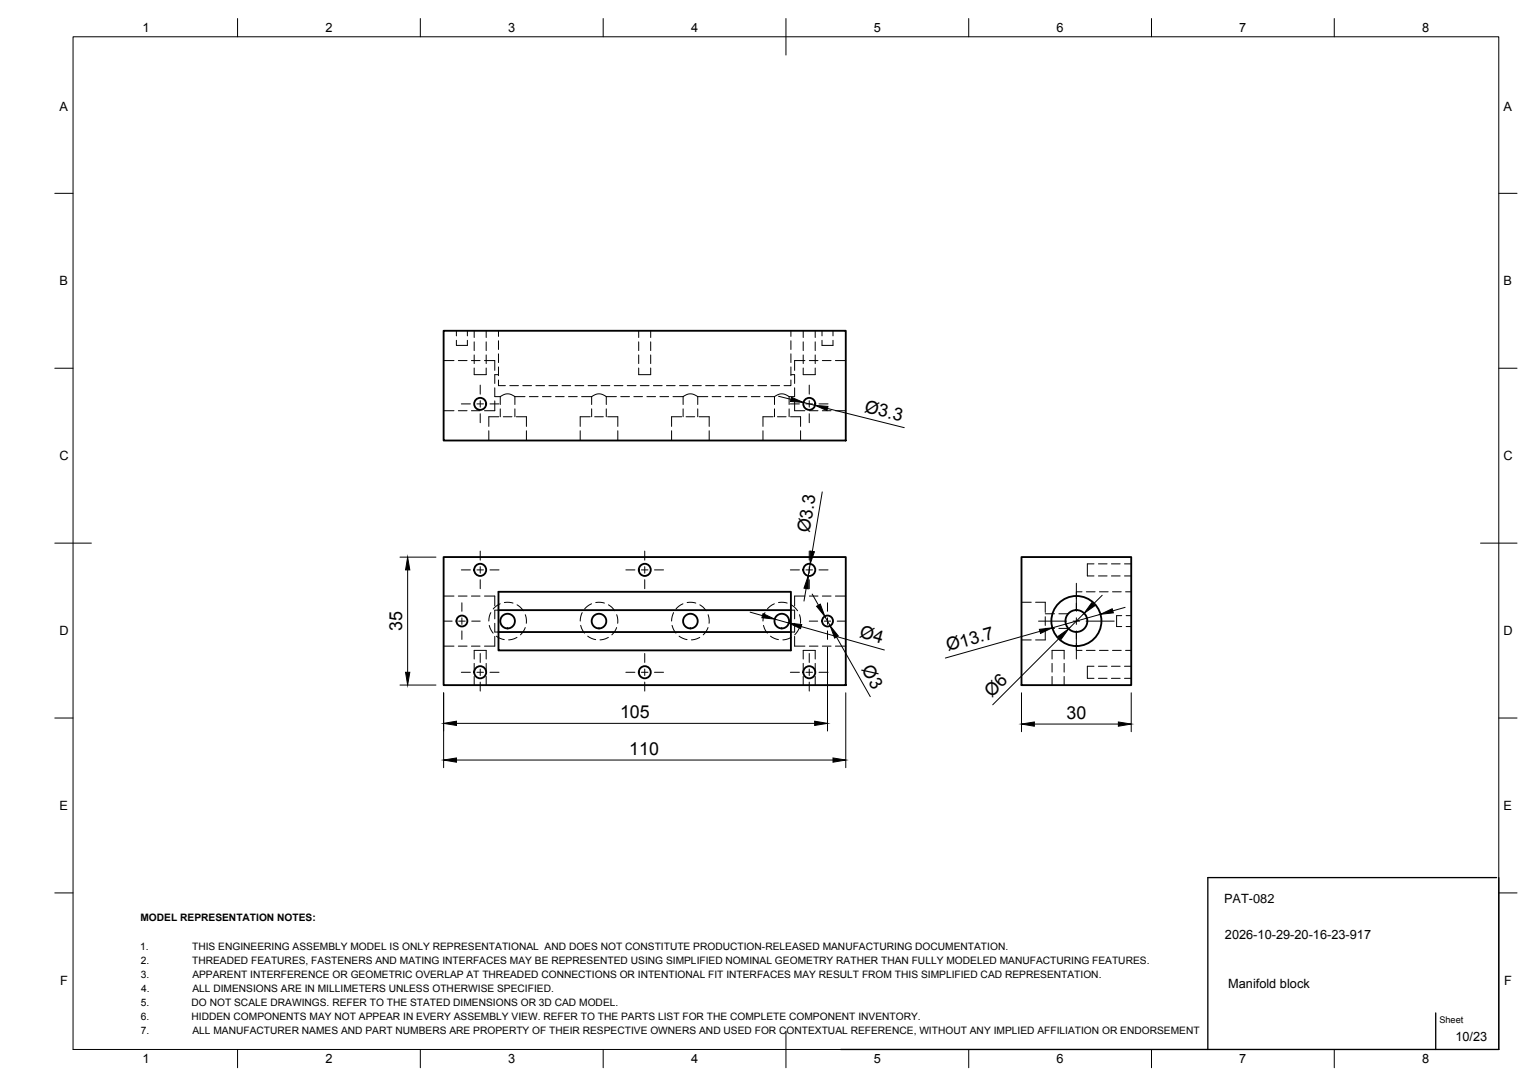
ISO-10303-21;
HEADER;
/* Generated by software containing ST-Developer
 * from STEP Tools, Inc. (www.steptools.com) 
 */

FILE_DESCRIPTION(
/* description */ ('PAT-082'),
/* implementation_level */ '2;1');

FILE_NAME(
/* name */ 'Manifold block.step',
/* time_stamp */ '2026-10-29T20:16:13-07:00',
/* author */ (''),
/* organization */ (''),
/* preprocessor_version */ 'ST-DEVELOPER v20.2',
/* originating_system */ 'Autodesk Translation Framework v15.17.0.0',
/* authorisation */ '');

FILE_SCHEMA (('AUTOMOTIVE_DESIGN { 1 0 10303 214 3 1 1 }'));
ENDSEC;

DATA;
#10=MECHANICAL_DESIGN_GEOMETRIC_PRESENTATION_REPRESENTATION('',(#248),#8266);
#185=B_SPLINE_CURVE_WITH_KNOTS('',3,(#7377,#7378,#7379,#7380,#7381,#7382,
#7383,#7384,#7385,#7386),.UNSPECIFIED.,.F.,.F.,(4,2,2,2,4),(0.,0.0789054703932598,
0.15781094078652,0.235848341776527,0.313885742766535),.UNSPECIFIED.);
#186=B_SPLINE_CURVE_WITH_KNOTS('',3,(#7388,#7389,#7390,#7391,#7392,#7393,
#7394,#7395,#7396,#7397),.UNSPECIFIED.,.F.,.F.,(4,2,2,2,4),(0.941657228299606,
1.01969462928961,1.09773203027962,1.17663750067288,1.25554297106614),
 .UNSPECIFIED.);
#187=B_SPLINE_CURVE_WITH_KNOTS('',3,(#7401,#7402,#7403,#7404,#7405,#7406,
#7407,#7408,#7409,#7410,#7411,#7412,#7413,#7414,#7415,#7416,#7417,#7418),
 .UNSPECIFIED.,.F.,.F.,(4,2,2,2,2,2,2,2,4),(0.313885742766535,0.391923143756543,
0.469960544746551,0.548866015139811,0.627771485533071,0.70667695592633,
0.78558242631959,0.863619827309598,0.941657228299606),.UNSPECIFIED.);
#188=B_SPLINE_CURVE_WITH_KNOTS('',3,(#7429,#7430,#7431,#7432,#7433,#7434,
#7435,#7436,#7437,#7438),.UNSPECIFIED.,.F.,.F.,(4,2,2,2,4),(0.,0.0789054703932594,
0.157810940786519,0.235848341776527,0.313885742766535),.UNSPECIFIED.);
#189=B_SPLINE_CURVE_WITH_KNOTS('',3,(#7440,#7441,#7442,#7443,#7444,#7445,
#7446,#7447,#7448,#7449),.UNSPECIFIED.,.F.,.F.,(4,2,2,2,4),(0.941657228299605,
1.01969462928961,1.09773203027962,1.17663750067288,1.25554297106614),
 .UNSPECIFIED.);
#190=B_SPLINE_CURVE_WITH_KNOTS('',3,(#7453,#7454,#7455,#7456,#7457,#7458,
#7459,#7460,#7461,#7462,#7463,#7464,#7465,#7466,#7467,#7468,#7469,#7470),
 .UNSPECIFIED.,.F.,.F.,(4,2,2,2,2,2,2,2,4),(0.313885742766535,0.391923143756543,
0.46996054474655,0.54886601513981,0.62777148553307,0.70667695592633,0.785582426319589,
0.863619827309597,0.941657228299605),.UNSPECIFIED.);
#191=B_SPLINE_CURVE_WITH_KNOTS('',3,(#7481,#7482,#7483,#7484,#7485,#7486,
#7487,#7488,#7489,#7490),.UNSPECIFIED.,.F.,.F.,(4,2,2,2,4),(0.,0.0789054703932594,
0.157810940786519,0.235848341776527,0.313885742766535),.UNSPECIFIED.);
#192=B_SPLINE_CURVE_WITH_KNOTS('',3,(#7492,#7493,#7494,#7495,#7496,#7497,
#7498,#7499,#7500,#7501),.UNSPECIFIED.,.F.,.F.,(4,2,2,2,4),(0.941657228299605,
1.01969462928961,1.09773203027962,1.17663750067288,1.25554297106614),
 .UNSPECIFIED.);
#193=B_SPLINE_CURVE_WITH_KNOTS('',3,(#7505,#7506,#7507,#7508,#7509,#7510,
#7511,#7512,#7513,#7514,#7515,#7516,#7517,#7518,#7519,#7520,#7521,#7522),
 .UNSPECIFIED.,.F.,.F.,(4,2,2,2,2,2,2,2,4),(0.313885742766535,0.391923143756543,
0.46996054474655,0.54886601513981,0.62777148553307,0.70667695592633,0.785582426319589,
0.863619827309597,0.941657228299605),.UNSPECIFIED.);
#194=B_SPLINE_CURVE_WITH_KNOTS('',3,(#7533,#7534,#7535,#7536,#7537,#7538,
#7539,#7540,#7541,#7542),.UNSPECIFIED.,.F.,.F.,(4,2,2,2,4),(0.,0.0789054703932596,
0.157810940786519,0.235848341776527,0.313885742766535),.UNSPECIFIED.);
#195=B_SPLINE_CURVE_WITH_KNOTS('',3,(#7544,#7545,#7546,#7547,#7548,#7549,
#7550,#7551,#7552,#7553),.UNSPECIFIED.,.F.,.F.,(4,2,2,2,4),(0.941657228299606,
1.01969462928961,1.09773203027962,1.17663750067288,1.25554297106614),
 .UNSPECIFIED.);
#196=B_SPLINE_CURVE_WITH_KNOTS('',3,(#7557,#7558,#7559,#7560,#7561,#7562,
#7563,#7564,#7565,#7566,#7567,#7568,#7569,#7570,#7571,#7572,#7573,#7574),
 .UNSPECIFIED.,.F.,.F.,(4,2,2,2,2,2,2,2,4),(0.313885742766535,0.391923143756543,
0.469960544746551,0.548866015139811,0.62777148553307,0.70667695592633,0.78558242631959,
0.863619827309598,0.941657228299606),.UNSPECIFIED.);
#204=SHAPE_REPRESENTATION_RELATIONSHIP('SRR','None',#8366,#226);
#226=ADVANCED_BREP_SHAPE_REPRESENTATION('',(#270),#8250);
#248=STYLED_ITEM('',(#8516),#270);
#270=MANIFOLD_SOLID_BREP('Body1',#4588);
#352=FACE_BOUND('',#1028,.T.);
#353=FACE_BOUND('',#1031,.T.);
#354=FACE_BOUND('',#1035,.T.);
#355=FACE_BOUND('',#1039,.T.);
#356=FACE_BOUND('',#1043,.T.);
#357=FACE_BOUND('',#1047,.T.);
#358=FACE_BOUND('',#1055,.T.);
#359=FACE_BOUND('',#1058,.T.);
#360=FACE_BOUND('',#1060,.T.);
#361=FACE_BOUND('',#1061,.T.);
#362=FACE_BOUND('',#1063,.T.);
#363=FACE_BOUND('',#1065,.T.);
#364=FACE_BOUND('',#1066,.T.);
#365=FACE_BOUND('',#1067,.T.);
#366=FACE_BOUND('',#1068,.T.);
#367=FACE_BOUND('',#1070,.T.);
#368=FACE_BOUND('',#1071,.T.);
#369=FACE_BOUND('',#1072,.T.);
#370=FACE_BOUND('',#1073,.T.);
#371=FACE_BOUND('',#1074,.T.);
#372=FACE_BOUND('',#1075,.T.);
#373=FACE_BOUND('',#1076,.T.);
#374=FACE_BOUND('',#1077,.T.);
#375=FACE_BOUND('',#1078,.T.);
#459=PLANE('',#5043);
#460=PLANE('',#5047);
#461=PLANE('',#5051);
#462=PLANE('',#5055);
#463=PLANE('',#5059);
#464=PLANE('',#5063);
#465=PLANE('',#5067);
#466=PLANE('',#5071);
#467=PLANE('',#5075);
#468=PLANE('',#5079);
#469=PLANE('',#5083);
#470=PLANE('',#5088);
#471=PLANE('',#5095);
#472=PLANE('',#5101);
#473=PLANE('',#5107);
#474=PLANE('',#5113);
#475=PLANE('',#5114);
#476=PLANE('',#5115);
#477=PLANE('',#5117);
#478=PLANE('',#5118);
#479=PLANE('',#5119);
#480=PLANE('',#5121);
#481=PLANE('',#5123);
#482=PLANE('',#5124);
#483=PLANE('',#5125);
#484=PLANE('',#5126);
#485=PLANE('',#5127);
#486=PLANE('',#5128);
#666=FACE_OUTER_BOUND('',#1006,.T.);
#667=FACE_OUTER_BOUND('',#1007,.T.);
#668=FACE_OUTER_BOUND('',#1008,.T.);
#669=FACE_OUTER_BOUND('',#1009,.T.);
#670=FACE_OUTER_BOUND('',#1010,.T.);
#671=FACE_OUTER_BOUND('',#1011,.T.);
#672=FACE_OUTER_BOUND('',#1012,.T.);
#673=FACE_OUTER_BOUND('',#1013,.T.);
#674=FACE_OUTER_BOUND('',#1014,.T.);
#675=FACE_OUTER_BOUND('',#1015,.T.);
#676=FACE_OUTER_BOUND('',#1016,.T.);
#677=FACE_OUTER_BOUND('',#1017,.T.);
#678=FACE_OUTER_BOUND('',#1018,.T.);
#679=FACE_OUTER_BOUND('',#1019,.T.);
#680=FACE_OUTER_BOUND('',#1020,.T.);
#681=FACE_OUTER_BOUND('',#1021,.T.);
#682=FACE_OUTER_BOUND('',#1022,.T.);
#683=FACE_OUTER_BOUND('',#1023,.T.);
#684=FACE_OUTER_BOUND('',#1024,.T.);
#685=FACE_OUTER_BOUND('',#1025,.T.);
#686=FACE_OUTER_BOUND('',#1026,.T.);
#687=FACE_OUTER_BOUND('',#1027,.T.);
#688=FACE_OUTER_BOUND('',#1029,.T.);
#689=FACE_OUTER_BOUND('',#1030,.T.);
#690=FACE_OUTER_BOUND('',#1032,.T.);
#691=FACE_OUTER_BOUND('',#1033,.T.);
#692=FACE_OUTER_BOUND('',#1034,.T.);
#693=FACE_OUTER_BOUND('',#1036,.T.);
#694=FACE_OUTER_BOUND('',#1037,.T.);
#695=FACE_OUTER_BOUND('',#1038,.T.);
#696=FACE_OUTER_BOUND('',#1040,.T.);
#697=FACE_OUTER_BOUND('',#1041,.T.);
#698=FACE_OUTER_BOUND('',#1042,.T.);
#699=FACE_OUTER_BOUND('',#1044,.T.);
#700=FACE_OUTER_BOUND('',#1045,.T.);
#701=FACE_OUTER_BOUND('',#1046,.T.);
#702=FACE_OUTER_BOUND('',#1048,.T.);
#703=FACE_OUTER_BOUND('',#1049,.T.);
#704=FACE_OUTER_BOUND('',#1050,.T.);
#705=FACE_OUTER_BOUND('',#1051,.T.);
#706=FACE_OUTER_BOUND('',#1052,.T.);
#707=FACE_OUTER_BOUND('',#1053,.T.);
#708=FACE_OUTER_BOUND('',#1054,.T.);
#709=FACE_OUTER_BOUND('',#1056,.T.);
#710=FACE_OUTER_BOUND('',#1057,.T.);
#711=FACE_OUTER_BOUND('',#1059,.T.);
#712=FACE_OUTER_BOUND('',#1062,.T.);
#713=FACE_OUTER_BOUND('',#1064,.T.);
#714=FACE_OUTER_BOUND('',#1069,.T.);
#1006=EDGE_LOOP('',(#3542,#3543,#3544,#3545));
#1007=EDGE_LOOP('',(#3546));
#1008=EDGE_LOOP('',(#3547,#3548,#3549,#3550));
#1009=EDGE_LOOP('',(#3551));
#1010=EDGE_LOOP('',(#3552,#3553,#3554,#3555));
#1011=EDGE_LOOP('',(#3556));
#1012=EDGE_LOOP('',(#3557,#3558,#3559,#3560));
#1013=EDGE_LOOP('',(#3561));
#1014=EDGE_LOOP('',(#3562,#3563,#3564,#3565));
#1015=EDGE_LOOP('',(#3566));
#1016=EDGE_LOOP('',(#3567,#3568,#3569,#3570));
#1017=EDGE_LOOP('',(#3571));
#1018=EDGE_LOOP('',(#3572,#3573,#3574,#3575));
#1019=EDGE_LOOP('',(#3576));
#1020=EDGE_LOOP('',(#3577,#3578,#3579,#3580));
#1021=EDGE_LOOP('',(#3581));
#1022=EDGE_LOOP('',(#3582,#3583,#3584,#3585));
#1023=EDGE_LOOP('',(#3586));
#1024=EDGE_LOOP('',(#3587,#3588,#3589,#3590));
#1025=EDGE_LOOP('',(#3591));
#1026=EDGE_LOOP('',(#3592,#3593,#3594,#3595));
#1027=EDGE_LOOP('',(#3596));
#1028=EDGE_LOOP('',(#3597));
#1029=EDGE_LOOP('',(#3598,#3599,#3600,#3601));
#1030=EDGE_LOOP('',(#3602));
#1031=EDGE_LOOP('',(#3603));
#1032=EDGE_LOOP('',(#3604,#3605,#3606,#3607,#3608,#3609));
#1033=EDGE_LOOP('',(#3610,#3611,#3612,#3613));
#1034=EDGE_LOOP('',(#3614));
#1035=EDGE_LOOP('',(#3615));
#1036=EDGE_LOOP('',(#3616,#3617,#3618,#3619,#3620,#3621));
#1037=EDGE_LOOP('',(#3622,#3623,#3624,#3625));
#1038=EDGE_LOOP('',(#3626));
#1039=EDGE_LOOP('',(#3627));
#1040=EDGE_LOOP('',(#3628,#3629,#3630,#3631,#3632,#3633));
#1041=EDGE_LOOP('',(#3634,#3635,#3636,#3637));
#1042=EDGE_LOOP('',(#3638));
#1043=EDGE_LOOP('',(#3639));
#1044=EDGE_LOOP('',(#3640,#3641,#3642,#3643,#3644,#3645));
#1045=EDGE_LOOP('',(#3646,#3647,#3648,#3649));
#1046=EDGE_LOOP('',(#3650));
#1047=EDGE_LOOP('',(#3651));
#1048=EDGE_LOOP('',(#3652,#3653,#3654,#3655));
#1049=EDGE_LOOP('',(#3656,#3657,#3658,#3659,#3660,#3661));
#1050=EDGE_LOOP('',(#3662,#3663,#3664,#3665));
#1051=EDGE_LOOP('',(#3666,#3667,#3668,#3669));
#1052=EDGE_LOOP('',(#3670,#3671,#3672,#3673,#3674,#3675));
#1053=EDGE_LOOP('',(#3676,#3677,#3678,#3679));
#1054=EDGE_LOOP('',(#3680,#3681,#3682,#3683,#3684,#3685,#3686,#3687,#3688,
#3689,#3690,#3691,#3692,#3693,#3694,#3695,#3696,#3697,#3698,#3699,#3700,
#3701,#3702,#3703));
#1055=EDGE_LOOP('',(#3704,#3705,#3706,#3707));
#1056=EDGE_LOOP('',(#3708,#3709,#3710,#3711));
#1057=EDGE_LOOP('',(#3712,#3713,#3714,#3715));
#1058=EDGE_LOOP('',(#3716));
#1059=EDGE_LOOP('',(#3717,#3718,#3719,#3720));
#1060=EDGE_LOOP('',(#3721));
#1061=EDGE_LOOP('',(#3722));
#1062=EDGE_LOOP('',(#3723,#3724,#3725,#3726));
#1063=EDGE_LOOP('',(#3727));
#1064=EDGE_LOOP('',(#3728,#3729,#3730,#3731));
#1065=EDGE_LOOP('',(#3732));
#1066=EDGE_LOOP('',(#3733));
#1067=EDGE_LOOP('',(#3734));
#1068=EDGE_LOOP('',(#3735));
#1069=EDGE_LOOP('',(#3736,#3737,#3738,#3739));
#1070=EDGE_LOOP('',(#3740));
#1071=EDGE_LOOP('',(#3741,#3742,#3743,#3744));
#1072=EDGE_LOOP('',(#3745));
#1073=EDGE_LOOP('',(#3746));
#1074=EDGE_LOOP('',(#3747));
#1075=EDGE_LOOP('',(#3748));
#1076=EDGE_LOOP('',(#3749));
#1077=EDGE_LOOP('',(#3750));
#1078=EDGE_LOOP('',(#3751));
#1375=LINE('',#7290,#1730);
#1376=LINE('',#7297,#1731);
#1377=LINE('',#7304,#1732);
#1378=LINE('',#7311,#1733);
#1379=LINE('',#7318,#1734);
#1380=LINE('',#7325,#1735);
#1381=LINE('',#7332,#1736);
#1382=LINE('',#7339,#1737);
#1383=LINE('',#7346,#1738);
#1384=LINE('',#7353,#1739);
#1385=LINE('',#7360,#1740);
#1386=LINE('',#7369,#1741);
#1387=LINE('',#7399,#1742);
#1388=LINE('',#7423,#1743);
#1389=LINE('',#7451,#1744);
#1390=LINE('',#7475,#1745);
#1391=LINE('',#7503,#1746);
#1392=LINE('',#7527,#1747);
#1393=LINE('',#7555,#1748);
#1394=LINE('',#7579,#1749);
#1395=LINE('',#7585,#1750);
#1396=LINE('',#7587,#1751);
#1397=LINE('',#7589,#1752);
#1398=LINE('',#7590,#1753);
#1399=LINE('',#7593,#1754);
#1400=LINE('',#7595,#1755);
#1401=LINE('',#7599,#1756);
#1402=LINE('',#7600,#1757);
#1403=LINE('',#7603,#1758);
#1404=LINE('',#7604,#1759);
#1405=LINE('',#7607,#1760);
#1406=LINE('',#7609,#1761);
#1407=LINE('',#7610,#1762);
#1408=LINE('',#7612,#1763);
#1409=LINE('',#7614,#1764);
#1410=LINE('',#7617,#1765);
#1411=LINE('',#7619,#1766);
#1412=LINE('',#7620,#1767);
#1413=LINE('',#7621,#1768);
#1414=LINE('',#7622,#1769);
#1415=LINE('',#7623,#1770);
#1416=LINE('',#7627,#1771);
#1417=LINE('',#7629,#1772);
#1418=LINE('',#7631,#1773);
#1419=LINE('',#7632,#1774);
#1420=LINE('',#7635,#1775);
#1421=LINE('',#7637,#1776);
#1422=LINE('',#7638,#1777);
#1423=LINE('',#7641,#1778);
#1424=LINE('',#7643,#1779);
#1425=LINE('',#7644,#1780);
#1426=LINE('',#7646,#1781);
#1427=LINE('',#7647,#1782);
#1730=VECTOR('',#5908,0.165);
#1731=VECTOR('',#5917,0.165);
#1732=VECTOR('',#5926,0.15);
#1733=VECTOR('',#5935,0.15);
#1734=VECTOR('',#5944,0.165);
#1735=VECTOR('',#5953,0.165);
#1736=VECTOR('',#5962,0.165);
#1737=VECTOR('',#5971,0.165);
#1738=VECTOR('',#5980,0.165);
#1739=VECTOR('',#5989,0.165);
#1740=VECTOR('',#5998,0.685);
#1741=VECTOR('',#6009,0.685);
#1742=VECTOR('',#6018,0.2);
#1743=VECTOR('',#6025,0.515);
#1744=VECTOR('',#6032,0.2);
#1745=VECTOR('',#6039,0.515);
#1746=VECTOR('',#6046,0.2);
#1747=VECTOR('',#6053,0.515);
#1748=VECTOR('',#6060,0.2);
#1749=VECTOR('',#6067,0.515);
#1750=VECTOR('',#6074,1.);
#1751=VECTOR('',#6075,1.);
#1752=VECTOR('',#6076,1.);
#1753=VECTOR('',#6077,1.);
#1754=VECTOR('',#6080,1.);
#1755=VECTOR('',#6081,1.);
#1756=VECTOR('',#6084,1.);
#1757=VECTOR('',#6085,1.);
#1758=VECTOR('',#6088,1.);
#1759=VECTOR('',#6089,1.);
#1760=VECTOR('',#6092,1.);
#1761=VECTOR('',#6093,1.);
#1762=VECTOR('',#6094,1.);
#1763=VECTOR('',#6097,1.);
#1764=VECTOR('',#6098,1.);
#1765=VECTOR('',#6103,1.);
#1766=VECTOR('',#6106,0.3);
#1767=VECTOR('',#6107,0.3);
#1768=VECTOR('',#6108,0.3);
#1769=VECTOR('',#6109,0.3);
#1770=VECTOR('',#6110,0.3);
#1771=VECTOR('',#6113,1.);
#1772=VECTOR('',#6114,1.);
#1773=VECTOR('',#6115,1.);
#1774=VECTOR('',#6116,1.);
#1775=VECTOR('',#6119,1.);
#1776=VECTOR('',#6120,1.);
#1777=VECTOR('',#6121,1.);
#1778=VECTOR('',#6124,1.);
#1779=VECTOR('',#6125,1.);
#1780=VECTOR('',#6126,1.);
#1781=VECTOR('',#6129,1.);
#1782=VECTOR('',#6130,1.);
#2033=CIRCLE('',#5041,0.165);
#2034=CIRCLE('',#5042,0.165);
#2035=CIRCLE('',#5045,0.165);
#2036=CIRCLE('',#5046,0.165);
#2037=CIRCLE('',#5049,0.15);
#2038=CIRCLE('',#5050,0.15);
#2039=CIRCLE('',#5053,0.15);
#2040=CIRCLE('',#5054,0.15);
#2041=CIRCLE('',#5057,0.165);
#2042=CIRCLE('',#5058,0.165);
#2043=CIRCLE('',#5061,0.165);
#2044=CIRCLE('',#5062,0.165);
#2045=CIRCLE('',#5065,0.165);
#2046=CIRCLE('',#5066,0.165);
#2047=CIRCLE('',#5069,0.165);
#2048=CIRCLE('',#5070,0.165);
#2049=CIRCLE('',#5073,0.165);
#2050=CIRCLE('',#5074,0.165);
#2051=CIRCLE('',#5077,0.165);
#2052=CIRCLE('',#5078,0.165);
#2053=CIRCLE('',#5081,0.685);
#2054=CIRCLE('',#5082,0.685);
#2055=CIRCLE('',#5084,0.3);
#2056=CIRCLE('',#5086,0.685);
#2057=CIRCLE('',#5087,0.685);
#2058=CIRCLE('',#5089,0.3);
#2059=CIRCLE('',#5091,0.2);
#2060=CIRCLE('',#5093,0.515);
#2061=CIRCLE('',#5094,0.515);
#2062=CIRCLE('',#5097,0.2);
#2063=CIRCLE('',#5099,0.515);
#2064=CIRCLE('',#5100,0.515);
#2065=CIRCLE('',#5103,0.2);
#2066=CIRCLE('',#5105,0.515);
#2067=CIRCLE('',#5106,0.515);
#2068=CIRCLE('',#5109,0.2);
#2069=CIRCLE('',#5111,0.515);
#2070=CIRCLE('',#5112,0.515);
#2071=CIRCLE('',#5116,0.3);
#2072=CIRCLE('',#5120,0.3);
#2297=VERTEX_POINT('',#7287);
#2298=VERTEX_POINT('',#7289);
#2299=VERTEX_POINT('',#7294);
#2300=VERTEX_POINT('',#7296);
#2301=VERTEX_POINT('',#7301);
#2302=VERTEX_POINT('',#7303);
#2303=VERTEX_POINT('',#7308);
#2304=VERTEX_POINT('',#7310);
#2305=VERTEX_POINT('',#7315);
#2306=VERTEX_POINT('',#7317);
#2307=VERTEX_POINT('',#7322);
#2308=VERTEX_POINT('',#7324);
#2309=VERTEX_POINT('',#7329);
#2310=VERTEX_POINT('',#7331);
#2311=VERTEX_POINT('',#7336);
#2312=VERTEX_POINT('',#7338);
#2313=VERTEX_POINT('',#7343);
#2314=VERTEX_POINT('',#7345);
#2315=VERTEX_POINT('',#7350);
#2316=VERTEX_POINT('',#7352);
#2317=VERTEX_POINT('',#7357);
#2318=VERTEX_POINT('',#7359);
#2319=VERTEX_POINT('',#7363);
#2320=VERTEX_POINT('',#7366);
#2321=VERTEX_POINT('',#7368);
#2322=VERTEX_POINT('',#7372);
#2323=VERTEX_POINT('',#7375);
#2324=VERTEX_POINT('',#7376);
#2325=VERTEX_POINT('',#7387);
#2326=VERTEX_POINT('',#7398);
#2327=VERTEX_POINT('',#7420);
#2328=VERTEX_POINT('',#7422);
#2329=VERTEX_POINT('',#7427);
#2330=VERTEX_POINT('',#7428);
#2331=VERTEX_POINT('',#7439);
#2332=VERTEX_POINT('',#7450);
#2333=VERTEX_POINT('',#7472);
#2334=VERTEX_POINT('',#7474);
#2335=VERTEX_POINT('',#7479);
#2336=VERTEX_POINT('',#7480);
#2337=VERTEX_POINT('',#7491);
#2338=VERTEX_POINT('',#7502);
#2339=VERTEX_POINT('',#7524);
#2340=VERTEX_POINT('',#7526);
#2341=VERTEX_POINT('',#7531);
#2342=VERTEX_POINT('',#7532);
#2343=VERTEX_POINT('',#7543);
#2344=VERTEX_POINT('',#7554);
#2345=VERTEX_POINT('',#7576);
#2346=VERTEX_POINT('',#7578);
#2347=VERTEX_POINT('',#7583);
#2348=VERTEX_POINT('',#7584);
#2349=VERTEX_POINT('',#7586);
#2350=VERTEX_POINT('',#7588);
#2351=VERTEX_POINT('',#7592);
#2352=VERTEX_POINT('',#7594);
#2353=VERTEX_POINT('',#7596);
#2354=VERTEX_POINT('',#7598);
#2355=VERTEX_POINT('',#7602);
#2356=VERTEX_POINT('',#7606);
#2357=VERTEX_POINT('',#7608);
#2358=VERTEX_POINT('',#7613);
#2359=VERTEX_POINT('',#7625);
#2360=VERTEX_POINT('',#7626);
#2361=VERTEX_POINT('',#7628);
#2362=VERTEX_POINT('',#7630);
#2363=VERTEX_POINT('',#7634);
#2364=VERTEX_POINT('',#7636);
#2365=VERTEX_POINT('',#7640);
#2366=VERTEX_POINT('',#7642);
#2747=EDGE_CURVE('',#2297,#2297,#2033,.T.);
#2748=EDGE_CURVE('',#2297,#2298,#1375,.T.);
#2749=EDGE_CURVE('',#2298,#2298,#2034,.T.);
#2750=EDGE_CURVE('',#2299,#2299,#2035,.T.);
#2751=EDGE_CURVE('',#2299,#2300,#1376,.T.);
#2752=EDGE_CURVE('',#2300,#2300,#2036,.T.);
#2753=EDGE_CURVE('',#2301,#2301,#2037,.T.);
#2754=EDGE_CURVE('',#2301,#2302,#1377,.T.);
#2755=EDGE_CURVE('',#2302,#2302,#2038,.T.);
#2756=EDGE_CURVE('',#2303,#2303,#2039,.T.);
#2757=EDGE_CURVE('',#2303,#2304,#1378,.T.);
#2758=EDGE_CURVE('',#2304,#2304,#2040,.T.);
#2759=EDGE_CURVE('',#2305,#2305,#2041,.T.);
#2760=EDGE_CURVE('',#2305,#2306,#1379,.T.);
#2761=EDGE_CURVE('',#2306,#2306,#2042,.T.);
#2762=EDGE_CURVE('',#2307,#2307,#2043,.T.);
#2763=EDGE_CURVE('',#2307,#2308,#1380,.T.);
#2764=EDGE_CURVE('',#2308,#2308,#2044,.T.);
#2765=EDGE_CURVE('',#2309,#2309,#2045,.T.);
#2766=EDGE_CURVE('',#2309,#2310,#1381,.T.);
#2767=EDGE_CURVE('',#2310,#2310,#2046,.T.);
#2768=EDGE_CURVE('',#2311,#2311,#2047,.T.);
#2769=EDGE_CURVE('',#2311,#2312,#1382,.T.);
#2770=EDGE_CURVE('',#2312,#2312,#2048,.T.);
#2771=EDGE_CURVE('',#2313,#2313,#2049,.T.);
#2772=EDGE_CURVE('',#2313,#2314,#1383,.T.);
#2773=EDGE_CURVE('',#2314,#2314,#2050,.T.);
#2774=EDGE_CURVE('',#2315,#2315,#2051,.T.);
#2775=EDGE_CURVE('',#2315,#2316,#1384,.T.);
#2776=EDGE_CURVE('',#2316,#2316,#2052,.T.);
#2777=EDGE_CURVE('',#2317,#2317,#2053,.T.);
#2778=EDGE_CURVE('',#2317,#2318,#1385,.T.);
#2779=EDGE_CURVE('',#2318,#2318,#2054,.T.);
#2780=EDGE_CURVE('',#2319,#2319,#2055,.T.);
#2781=EDGE_CURVE('',#2320,#2320,#2056,.T.);
#2782=EDGE_CURVE('',#2320,#2321,#1386,.T.);
#2783=EDGE_CURVE('',#2321,#2321,#2057,.T.);
#2784=EDGE_CURVE('',#2322,#2322,#2058,.T.);
#2785=EDGE_CURVE('',#2323,#2324,#185,.T.);
#2786=EDGE_CURVE('',#2325,#2323,#186,.T.);
#2787=EDGE_CURVE('',#2325,#2326,#1387,.T.);
#2788=EDGE_CURVE('',#2326,#2326,#2059,.T.);
#2789=EDGE_CURVE('',#2324,#2325,#187,.T.);
#2790=EDGE_CURVE('',#2327,#2327,#2060,.T.);
#2791=EDGE_CURVE('',#2327,#2328,#1388,.T.);
#2792=EDGE_CURVE('',#2328,#2328,#2061,.T.);
#2793=EDGE_CURVE('',#2329,#2330,#188,.T.);
#2794=EDGE_CURVE('',#2331,#2329,#189,.T.);
#2795=EDGE_CURVE('',#2331,#2332,#1389,.T.);
#2796=EDGE_CURVE('',#2332,#2332,#2062,.T.);
#2797=EDGE_CURVE('',#2330,#2331,#190,.T.);
#2798=EDGE_CURVE('',#2333,#2333,#2063,.T.);
#2799=EDGE_CURVE('',#2333,#2334,#1390,.T.);
#2800=EDGE_CURVE('',#2334,#2334,#2064,.T.);
#2801=EDGE_CURVE('',#2335,#2336,#191,.T.);
#2802=EDGE_CURVE('',#2337,#2335,#192,.T.);
#2803=EDGE_CURVE('',#2337,#2338,#1391,.T.);
#2804=EDGE_CURVE('',#2338,#2338,#2065,.T.);
#2805=EDGE_CURVE('',#2336,#2337,#193,.T.);
#2806=EDGE_CURVE('',#2339,#2339,#2066,.T.);
#2807=EDGE_CURVE('',#2339,#2340,#1392,.T.);
#2808=EDGE_CURVE('',#2340,#2340,#2067,.T.);
#2809=EDGE_CURVE('',#2341,#2342,#194,.T.);
#2810=EDGE_CURVE('',#2343,#2341,#195,.T.);
#2811=EDGE_CURVE('',#2343,#2344,#1393,.T.);
#2812=EDGE_CURVE('',#2344,#2344,#2068,.T.);
#2813=EDGE_CURVE('',#2342,#2343,#196,.T.);
#2814=EDGE_CURVE('',#2345,#2345,#2069,.T.);
#2815=EDGE_CURVE('',#2345,#2346,#1394,.T.);
#2816=EDGE_CURVE('',#2346,#2346,#2070,.T.);
#2817=EDGE_CURVE('',#2347,#2348,#1395,.T.);
#2818=EDGE_CURVE('',#2347,#2349,#1396,.T.);
#2819=EDGE_CURVE('',#2349,#2350,#1397,.T.);
#2820=EDGE_CURVE('',#2348,#2350,#1398,.T.);
#2821=EDGE_CURVE('',#2348,#2351,#1399,.T.);
#2822=EDGE_CURVE('',#2350,#2352,#1400,.T.);
#2823=EDGE_CURVE('',#2353,#2352,#2071,.T.);
#2824=EDGE_CURVE('',#2353,#2354,#1401,.T.);
#2825=EDGE_CURVE('',#2351,#2354,#1402,.T.);
#2826=EDGE_CURVE('',#2352,#2355,#1403,.T.);
#2827=EDGE_CURVE('',#2355,#2349,#1404,.T.);
#2828=EDGE_CURVE('',#2351,#2356,#1405,.T.);
#2829=EDGE_CURVE('',#2354,#2357,#1406,.T.);
#2830=EDGE_CURVE('',#2356,#2357,#1407,.T.);
#2831=EDGE_CURVE('',#2356,#2347,#1408,.T.);
#2832=EDGE_CURVE('',#2357,#2358,#1409,.T.);
#2833=EDGE_CURVE('',#2355,#2358,#2072,.T.);
#2834=EDGE_CURVE('',#2358,#2353,#1410,.T.);
#2835=EDGE_CURVE('',#2322,#2343,#1411,.T.);
#2836=EDGE_CURVE('',#2342,#2337,#1412,.T.);
#2837=EDGE_CURVE('',#2336,#2331,#1413,.T.);
#2838=EDGE_CURVE('',#2330,#2325,#1414,.T.);
#2839=EDGE_CURVE('',#2324,#2319,#1415,.T.);
#2840=EDGE_CURVE('',#2359,#2360,#1416,.T.);
#2841=EDGE_CURVE('',#2360,#2361,#1417,.T.);
#2842=EDGE_CURVE('',#2362,#2361,#1418,.T.);
#2843=EDGE_CURVE('',#2359,#2362,#1419,.T.);
#2844=EDGE_CURVE('',#2363,#2359,#1420,.T.);
#2845=EDGE_CURVE('',#2364,#2362,#1421,.T.);
#2846=EDGE_CURVE('',#2363,#2364,#1422,.T.);
#2847=EDGE_CURVE('',#2365,#2363,#1423,.T.);
#2848=EDGE_CURVE('',#2366,#2364,#1424,.T.);
#2849=EDGE_CURVE('',#2365,#2366,#1425,.T.);
#2850=EDGE_CURVE('',#2360,#2365,#1426,.T.);
#2851=EDGE_CURVE('',#2361,#2366,#1427,.T.);
#3542=ORIENTED_EDGE('',*,*,#2747,.F.);
#3543=ORIENTED_EDGE('',*,*,#2748,.T.);
#3544=ORIENTED_EDGE('',*,*,#2749,.T.);
#3545=ORIENTED_EDGE('',*,*,#2748,.F.);
#3546=ORIENTED_EDGE('',*,*,#2749,.F.);
#3547=ORIENTED_EDGE('',*,*,#2750,.F.);
#3548=ORIENTED_EDGE('',*,*,#2751,.T.);
#3549=ORIENTED_EDGE('',*,*,#2752,.T.);
#3550=ORIENTED_EDGE('',*,*,#2751,.F.);
#3551=ORIENTED_EDGE('',*,*,#2752,.F.);
#3552=ORIENTED_EDGE('',*,*,#2753,.F.);
#3553=ORIENTED_EDGE('',*,*,#2754,.T.);
#3554=ORIENTED_EDGE('',*,*,#2755,.T.);
#3555=ORIENTED_EDGE('',*,*,#2754,.F.);
#3556=ORIENTED_EDGE('',*,*,#2755,.F.);
#3557=ORIENTED_EDGE('',*,*,#2756,.F.);
#3558=ORIENTED_EDGE('',*,*,#2757,.T.);
#3559=ORIENTED_EDGE('',*,*,#2758,.T.);
#3560=ORIENTED_EDGE('',*,*,#2757,.F.);
#3561=ORIENTED_EDGE('',*,*,#2758,.F.);
#3562=ORIENTED_EDGE('',*,*,#2759,.F.);
#3563=ORIENTED_EDGE('',*,*,#2760,.T.);
#3564=ORIENTED_EDGE('',*,*,#2761,.T.);
#3565=ORIENTED_EDGE('',*,*,#2760,.F.);
#3566=ORIENTED_EDGE('',*,*,#2761,.F.);
#3567=ORIENTED_EDGE('',*,*,#2762,.F.);
#3568=ORIENTED_EDGE('',*,*,#2763,.T.);
#3569=ORIENTED_EDGE('',*,*,#2764,.T.);
#3570=ORIENTED_EDGE('',*,*,#2763,.F.);
#3571=ORIENTED_EDGE('',*,*,#2764,.F.);
#3572=ORIENTED_EDGE('',*,*,#2765,.F.);
#3573=ORIENTED_EDGE('',*,*,#2766,.T.);
#3574=ORIENTED_EDGE('',*,*,#2767,.T.);
#3575=ORIENTED_EDGE('',*,*,#2766,.F.);
#3576=ORIENTED_EDGE('',*,*,#2767,.F.);
#3577=ORIENTED_EDGE('',*,*,#2768,.F.);
#3578=ORIENTED_EDGE('',*,*,#2769,.T.);
#3579=ORIENTED_EDGE('',*,*,#2770,.T.);
#3580=ORIENTED_EDGE('',*,*,#2769,.F.);
#3581=ORIENTED_EDGE('',*,*,#2770,.F.);
#3582=ORIENTED_EDGE('',*,*,#2771,.F.);
#3583=ORIENTED_EDGE('',*,*,#2772,.T.);
#3584=ORIENTED_EDGE('',*,*,#2773,.T.);
#3585=ORIENTED_EDGE('',*,*,#2772,.F.);
#3586=ORIENTED_EDGE('',*,*,#2773,.F.);
#3587=ORIENTED_EDGE('',*,*,#2774,.F.);
#3588=ORIENTED_EDGE('',*,*,#2775,.T.);
#3589=ORIENTED_EDGE('',*,*,#2776,.T.);
#3590=ORIENTED_EDGE('',*,*,#2775,.F.);
#3591=ORIENTED_EDGE('',*,*,#2776,.F.);
#3592=ORIENTED_EDGE('',*,*,#2777,.F.);
#3593=ORIENTED_EDGE('',*,*,#2778,.T.);
#3594=ORIENTED_EDGE('',*,*,#2779,.F.);
#3595=ORIENTED_EDGE('',*,*,#2778,.F.);
#3596=ORIENTED_EDGE('',*,*,#2777,.T.);
#3597=ORIENTED_EDGE('',*,*,#2780,.F.);
#3598=ORIENTED_EDGE('',*,*,#2781,.F.);
#3599=ORIENTED_EDGE('',*,*,#2782,.T.);
#3600=ORIENTED_EDGE('',*,*,#2783,.T.);
#3601=ORIENTED_EDGE('',*,*,#2782,.F.);
#3602=ORIENTED_EDGE('',*,*,#2783,.F.);
#3603=ORIENTED_EDGE('',*,*,#2784,.F.);
#3604=ORIENTED_EDGE('',*,*,#2785,.F.);
#3605=ORIENTED_EDGE('',*,*,#2786,.F.);
#3606=ORIENTED_EDGE('',*,*,#2787,.T.);
#3607=ORIENTED_EDGE('',*,*,#2788,.F.);
#3608=ORIENTED_EDGE('',*,*,#2787,.F.);
#3609=ORIENTED_EDGE('',*,*,#2789,.F.);
#3610=ORIENTED_EDGE('',*,*,#2790,.F.);
#3611=ORIENTED_EDGE('',*,*,#2791,.T.);
#3612=ORIENTED_EDGE('',*,*,#2792,.F.);
#3613=ORIENTED_EDGE('',*,*,#2791,.F.);
#3614=ORIENTED_EDGE('',*,*,#2790,.T.);
#3615=ORIENTED_EDGE('',*,*,#2788,.T.);
#3616=ORIENTED_EDGE('',*,*,#2793,.F.);
#3617=ORIENTED_EDGE('',*,*,#2794,.F.);
#3618=ORIENTED_EDGE('',*,*,#2795,.T.);
#3619=ORIENTED_EDGE('',*,*,#2796,.F.);
#3620=ORIENTED_EDGE('',*,*,#2795,.F.);
#3621=ORIENTED_EDGE('',*,*,#2797,.F.);
#3622=ORIENTED_EDGE('',*,*,#2798,.F.);
#3623=ORIENTED_EDGE('',*,*,#2799,.T.);
#3624=ORIENTED_EDGE('',*,*,#2800,.F.);
#3625=ORIENTED_EDGE('',*,*,#2799,.F.);
#3626=ORIENTED_EDGE('',*,*,#2798,.T.);
#3627=ORIENTED_EDGE('',*,*,#2796,.T.);
#3628=ORIENTED_EDGE('',*,*,#2801,.F.);
#3629=ORIENTED_EDGE('',*,*,#2802,.F.);
#3630=ORIENTED_EDGE('',*,*,#2803,.T.);
#3631=ORIENTED_EDGE('',*,*,#2804,.F.);
#3632=ORIENTED_EDGE('',*,*,#2803,.F.);
#3633=ORIENTED_EDGE('',*,*,#2805,.F.);
#3634=ORIENTED_EDGE('',*,*,#2806,.F.);
#3635=ORIENTED_EDGE('',*,*,#2807,.T.);
#3636=ORIENTED_EDGE('',*,*,#2808,.F.);
#3637=ORIENTED_EDGE('',*,*,#2807,.F.);
#3638=ORIENTED_EDGE('',*,*,#2806,.T.);
#3639=ORIENTED_EDGE('',*,*,#2804,.T.);
#3640=ORIENTED_EDGE('',*,*,#2809,.F.);
#3641=ORIENTED_EDGE('',*,*,#2810,.F.);
#3642=ORIENTED_EDGE('',*,*,#2811,.T.);
#3643=ORIENTED_EDGE('',*,*,#2812,.F.);
#3644=ORIENTED_EDGE('',*,*,#2811,.F.);
#3645=ORIENTED_EDGE('',*,*,#2813,.F.);
#3646=ORIENTED_EDGE('',*,*,#2814,.F.);
#3647=ORIENTED_EDGE('',*,*,#2815,.T.);
#3648=ORIENTED_EDGE('',*,*,#2816,.F.);
#3649=ORIENTED_EDGE('',*,*,#2815,.F.);
#3650=ORIENTED_EDGE('',*,*,#2814,.T.);
#3651=ORIENTED_EDGE('',*,*,#2812,.T.);
#3652=ORIENTED_EDGE('',*,*,#2817,.F.);
#3653=ORIENTED_EDGE('',*,*,#2818,.T.);
#3654=ORIENTED_EDGE('',*,*,#2819,.T.);
#3655=ORIENTED_EDGE('',*,*,#2820,.F.);
#3656=ORIENTED_EDGE('',*,*,#2821,.F.);
#3657=ORIENTED_EDGE('',*,*,#2820,.T.);
#3658=ORIENTED_EDGE('',*,*,#2822,.T.);
#3659=ORIENTED_EDGE('',*,*,#2823,.F.);
#3660=ORIENTED_EDGE('',*,*,#2824,.T.);
#3661=ORIENTED_EDGE('',*,*,#2825,.F.);
#3662=ORIENTED_EDGE('',*,*,#2826,.F.);
#3663=ORIENTED_EDGE('',*,*,#2822,.F.);
#3664=ORIENTED_EDGE('',*,*,#2819,.F.);
#3665=ORIENTED_EDGE('',*,*,#2827,.F.);
#3666=ORIENTED_EDGE('',*,*,#2828,.F.);
#3667=ORIENTED_EDGE('',*,*,#2825,.T.);
#3668=ORIENTED_EDGE('',*,*,#2829,.T.);
#3669=ORIENTED_EDGE('',*,*,#2830,.F.);
#3670=ORIENTED_EDGE('',*,*,#2831,.F.);
#3671=ORIENTED_EDGE('',*,*,#2830,.T.);
#3672=ORIENTED_EDGE('',*,*,#2832,.T.);
#3673=ORIENTED_EDGE('',*,*,#2833,.F.);
#3674=ORIENTED_EDGE('',*,*,#2827,.T.);
#3675=ORIENTED_EDGE('',*,*,#2818,.F.);
#3676=ORIENTED_EDGE('',*,*,#2834,.F.);
#3677=ORIENTED_EDGE('',*,*,#2832,.F.);
#3678=ORIENTED_EDGE('',*,*,#2829,.F.);
#3679=ORIENTED_EDGE('',*,*,#2824,.F.);
#3680=ORIENTED_EDGE('',*,*,#2784,.T.);
#3681=ORIENTED_EDGE('',*,*,#2835,.T.);
#3682=ORIENTED_EDGE('',*,*,#2810,.T.);
#3683=ORIENTED_EDGE('',*,*,#2809,.T.);
#3684=ORIENTED_EDGE('',*,*,#2836,.T.);
#3685=ORIENTED_EDGE('',*,*,#2802,.T.);
#3686=ORIENTED_EDGE('',*,*,#2801,.T.);
#3687=ORIENTED_EDGE('',*,*,#2837,.T.);
#3688=ORIENTED_EDGE('',*,*,#2794,.T.);
#3689=ORIENTED_EDGE('',*,*,#2793,.T.);
#3690=ORIENTED_EDGE('',*,*,#2838,.T.);
#3691=ORIENTED_EDGE('',*,*,#2786,.T.);
#3692=ORIENTED_EDGE('',*,*,#2785,.T.);
#3693=ORIENTED_EDGE('',*,*,#2839,.T.);
#3694=ORIENTED_EDGE('',*,*,#2780,.T.);
#3695=ORIENTED_EDGE('',*,*,#2839,.F.);
#3696=ORIENTED_EDGE('',*,*,#2789,.T.);
#3697=ORIENTED_EDGE('',*,*,#2838,.F.);
#3698=ORIENTED_EDGE('',*,*,#2797,.T.);
#3699=ORIENTED_EDGE('',*,*,#2837,.F.);
#3700=ORIENTED_EDGE('',*,*,#2805,.T.);
#3701=ORIENTED_EDGE('',*,*,#2836,.F.);
#3702=ORIENTED_EDGE('',*,*,#2813,.T.);
#3703=ORIENTED_EDGE('',*,*,#2835,.F.);
#3704=ORIENTED_EDGE('',*,*,#2833,.T.);
#3705=ORIENTED_EDGE('',*,*,#2834,.T.);
#3706=ORIENTED_EDGE('',*,*,#2823,.T.);
#3707=ORIENTED_EDGE('',*,*,#2826,.T.);
#3708=ORIENTED_EDGE('',*,*,#2840,.T.);
#3709=ORIENTED_EDGE('',*,*,#2841,.T.);
#3710=ORIENTED_EDGE('',*,*,#2842,.F.);
#3711=ORIENTED_EDGE('',*,*,#2843,.F.);
#3712=ORIENTED_EDGE('',*,*,#2844,.T.);
#3713=ORIENTED_EDGE('',*,*,#2843,.T.);
#3714=ORIENTED_EDGE('',*,*,#2845,.F.);
#3715=ORIENTED_EDGE('',*,*,#2846,.F.);
#3716=ORIENTED_EDGE('',*,*,#2779,.T.);
#3717=ORIENTED_EDGE('',*,*,#2847,.T.);
#3718=ORIENTED_EDGE('',*,*,#2846,.T.);
#3719=ORIENTED_EDGE('',*,*,#2848,.F.);
#3720=ORIENTED_EDGE('',*,*,#2849,.F.);
#3721=ORIENTED_EDGE('',*,*,#2747,.T.);
#3722=ORIENTED_EDGE('',*,*,#2750,.T.);
#3723=ORIENTED_EDGE('',*,*,#2850,.T.);
#3724=ORIENTED_EDGE('',*,*,#2849,.T.);
#3725=ORIENTED_EDGE('',*,*,#2851,.F.);
#3726=ORIENTED_EDGE('',*,*,#2841,.F.);
#3727=ORIENTED_EDGE('',*,*,#2781,.T.);
#3728=ORIENTED_EDGE('',*,*,#2851,.T.);
#3729=ORIENTED_EDGE('',*,*,#2848,.T.);
#3730=ORIENTED_EDGE('',*,*,#2845,.T.);
#3731=ORIENTED_EDGE('',*,*,#2842,.T.);
#3732=ORIENTED_EDGE('',*,*,#2792,.T.);
#3733=ORIENTED_EDGE('',*,*,#2800,.T.);
#3734=ORIENTED_EDGE('',*,*,#2808,.T.);
#3735=ORIENTED_EDGE('',*,*,#2816,.T.);
#3736=ORIENTED_EDGE('',*,*,#2850,.F.);
#3737=ORIENTED_EDGE('',*,*,#2840,.F.);
#3738=ORIENTED_EDGE('',*,*,#2844,.F.);
#3739=ORIENTED_EDGE('',*,*,#2847,.F.);
#3740=ORIENTED_EDGE('',*,*,#2756,.T.);
#3741=ORIENTED_EDGE('',*,*,#2828,.T.);
#3742=ORIENTED_EDGE('',*,*,#2831,.T.);
#3743=ORIENTED_EDGE('',*,*,#2817,.T.);
#3744=ORIENTED_EDGE('',*,*,#2821,.T.);
#3745=ORIENTED_EDGE('',*,*,#2774,.T.);
#3746=ORIENTED_EDGE('',*,*,#2771,.T.);
#3747=ORIENTED_EDGE('',*,*,#2768,.T.);
#3748=ORIENTED_EDGE('',*,*,#2765,.T.);
#3749=ORIENTED_EDGE('',*,*,#2762,.T.);
#3750=ORIENTED_EDGE('',*,*,#2759,.T.);
#3751=ORIENTED_EDGE('',*,*,#2753,.T.);
#4260=CYLINDRICAL_SURFACE('',#5040,0.165);
#4261=CYLINDRICAL_SURFACE('',#5044,0.165);
#4262=CYLINDRICAL_SURFACE('',#5048,0.15);
#4263=CYLINDRICAL_SURFACE('',#5052,0.15);
#4264=CYLINDRICAL_SURFACE('',#5056,0.165);
#4265=CYLINDRICAL_SURFACE('',#5060,0.165);
#4266=CYLINDRICAL_SURFACE('',#5064,0.165);
#4267=CYLINDRICAL_SURFACE('',#5068,0.165);
#4268=CYLINDRICAL_SURFACE('',#5072,0.165);
#4269=CYLINDRICAL_SURFACE('',#5076,0.165);
#4270=CYLINDRICAL_SURFACE('',#5080,0.685);
#4271=CYLINDRICAL_SURFACE('',#5085,0.685);
#4272=CYLINDRICAL_SURFACE('',#5090,0.2);
#4273=CYLINDRICAL_SURFACE('',#5092,0.515);
#4274=CYLINDRICAL_SURFACE('',#5096,0.2);
#4275=CYLINDRICAL_SURFACE('',#5098,0.515);
#4276=CYLINDRICAL_SURFACE('',#5102,0.2);
#4277=CYLINDRICAL_SURFACE('',#5104,0.515);
#4278=CYLINDRICAL_SURFACE('',#5108,0.2);
#4279=CYLINDRICAL_SURFACE('',#5110,0.515);
#4280=CYLINDRICAL_SURFACE('',#5122,0.3);
#4405=ADVANCED_FACE('',(#666),#4260,.F.);
#4406=ADVANCED_FACE('',(#667),#459,.F.);
#4407=ADVANCED_FACE('',(#668),#4261,.F.);
#4408=ADVANCED_FACE('',(#669),#460,.F.);
#4409=ADVANCED_FACE('',(#670),#4262,.F.);
#4410=ADVANCED_FACE('',(#671),#461,.F.);
#4411=ADVANCED_FACE('',(#672),#4263,.F.);
#4412=ADVANCED_FACE('',(#673),#462,.F.);
#4413=ADVANCED_FACE('',(#674),#4264,.F.);
#4414=ADVANCED_FACE('',(#675),#463,.F.);
#4415=ADVANCED_FACE('',(#676),#4265,.F.);
#4416=ADVANCED_FACE('',(#677),#464,.F.);
#4417=ADVANCED_FACE('',(#678),#4266,.F.);
#4418=ADVANCED_FACE('',(#679),#465,.F.);
#4419=ADVANCED_FACE('',(#680),#4267,.F.);
#4420=ADVANCED_FACE('',(#681),#466,.F.);
#4421=ADVANCED_FACE('',(#682),#4268,.F.);
#4422=ADVANCED_FACE('',(#683),#467,.F.);
#4423=ADVANCED_FACE('',(#684),#4269,.F.);
#4424=ADVANCED_FACE('',(#685),#468,.F.);
#4425=ADVANCED_FACE('',(#686),#4270,.F.);
#4426=ADVANCED_FACE('',(#687,#352),#469,.T.);
#4427=ADVANCED_FACE('',(#688),#4271,.F.);
#4428=ADVANCED_FACE('',(#689,#353),#470,.F.);
#4429=ADVANCED_FACE('',(#690),#4272,.F.);
#4430=ADVANCED_FACE('',(#691),#4273,.F.);
#4431=ADVANCED_FACE('',(#692,#354),#471,.T.);
#4432=ADVANCED_FACE('',(#693),#4274,.F.);
#4433=ADVANCED_FACE('',(#694),#4275,.F.);
#4434=ADVANCED_FACE('',(#695,#355),#472,.T.);
#4435=ADVANCED_FACE('',(#696),#4276,.F.);
#4436=ADVANCED_FACE('',(#697),#4277,.F.);
#4437=ADVANCED_FACE('',(#698,#356),#473,.T.);
#4438=ADVANCED_FACE('',(#699),#4278,.F.);
#4439=ADVANCED_FACE('',(#700),#4279,.F.);
#4440=ADVANCED_FACE('',(#701,#357),#474,.T.);
#4441=ADVANCED_FACE('',(#702),#475,.F.);
#4442=ADVANCED_FACE('',(#703),#476,.F.);
#4443=ADVANCED_FACE('',(#704),#477,.F.);
#4444=ADVANCED_FACE('',(#705),#478,.F.);
#4445=ADVANCED_FACE('',(#706),#479,.F.);
#4446=ADVANCED_FACE('',(#707),#480,.F.);
#4447=ADVANCED_FACE('',(#708,#358),#4280,.F.);
#4448=ADVANCED_FACE('',(#709),#481,.T.);
#4449=ADVANCED_FACE('',(#710,#359),#482,.T.);
#4450=ADVANCED_FACE('',(#711,#360,#361),#483,.T.);
#4451=ADVANCED_FACE('',(#712,#362),#484,.T.);
#4452=ADVANCED_FACE('',(#713,#363,#364,#365,#366),#485,.T.);
#4453=ADVANCED_FACE('',(#714,#367,#368,#369,#370,#371,#372,#373,#374,#375),
#486,.F.);
#4588=CLOSED_SHELL('',(#4405,#4406,#4407,#4408,#4409,#4410,#4411,#4412,
#4413,#4414,#4415,#4416,#4417,#4418,#4419,#4420,#4421,#4422,#4423,#4424,
#4425,#4426,#4427,#4428,#4429,#4430,#4431,#4432,#4433,#4434,#4435,#4436,
#4437,#4438,#4439,#4440,#4441,#4442,#4443,#4444,#4445,#4446,#4447,#4448,
#4449,#4450,#4451,#4452,#4453));
#5039=AXIS2_PLACEMENT_3D('',#7285,#5902,#5903);
#5040=AXIS2_PLACEMENT_3D('',#7286,#5904,#5905);
#5041=AXIS2_PLACEMENT_3D('',#7288,#5906,#5907);
#5042=AXIS2_PLACEMENT_3D('',#7291,#5909,#5910);
#5043=AXIS2_PLACEMENT_3D('',#7292,#5911,#5912);
#5044=AXIS2_PLACEMENT_3D('',#7293,#5913,#5914);
#5045=AXIS2_PLACEMENT_3D('',#7295,#5915,#5916);
#5046=AXIS2_PLACEMENT_3D('',#7298,#5918,#5919);
#5047=AXIS2_PLACEMENT_3D('',#7299,#5920,#5921);
#5048=AXIS2_PLACEMENT_3D('',#7300,#5922,#5923);
#5049=AXIS2_PLACEMENT_3D('',#7302,#5924,#5925);
#5050=AXIS2_PLACEMENT_3D('',#7305,#5927,#5928);
#5051=AXIS2_PLACEMENT_3D('',#7306,#5929,#5930);
#5052=AXIS2_PLACEMENT_3D('',#7307,#5931,#5932);
#5053=AXIS2_PLACEMENT_3D('',#7309,#5933,#5934);
#5054=AXIS2_PLACEMENT_3D('',#7312,#5936,#5937);
#5055=AXIS2_PLACEMENT_3D('',#7313,#5938,#5939);
#5056=AXIS2_PLACEMENT_3D('',#7314,#5940,#5941);
#5057=AXIS2_PLACEMENT_3D('',#7316,#5942,#5943);
#5058=AXIS2_PLACEMENT_3D('',#7319,#5945,#5946);
#5059=AXIS2_PLACEMENT_3D('',#7320,#5947,#5948);
#5060=AXIS2_PLACEMENT_3D('',#7321,#5949,#5950);
#5061=AXIS2_PLACEMENT_3D('',#7323,#5951,#5952);
#5062=AXIS2_PLACEMENT_3D('',#7326,#5954,#5955);
#5063=AXIS2_PLACEMENT_3D('',#7327,#5956,#5957);
#5064=AXIS2_PLACEMENT_3D('',#7328,#5958,#5959);
#5065=AXIS2_PLACEMENT_3D('',#7330,#5960,#5961);
#5066=AXIS2_PLACEMENT_3D('',#7333,#5963,#5964);
#5067=AXIS2_PLACEMENT_3D('',#7334,#5965,#5966);
#5068=AXIS2_PLACEMENT_3D('',#7335,#5967,#5968);
#5069=AXIS2_PLACEMENT_3D('',#7337,#5969,#5970);
#5070=AXIS2_PLACEMENT_3D('',#7340,#5972,#5973);
#5071=AXIS2_PLACEMENT_3D('',#7341,#5974,#5975);
#5072=AXIS2_PLACEMENT_3D('',#7342,#5976,#5977);
#5073=AXIS2_PLACEMENT_3D('',#7344,#5978,#5979);
#5074=AXIS2_PLACEMENT_3D('',#7347,#5981,#5982);
#5075=AXIS2_PLACEMENT_3D('',#7348,#5983,#5984);
#5076=AXIS2_PLACEMENT_3D('',#7349,#5985,#5986);
#5077=AXIS2_PLACEMENT_3D('',#7351,#5987,#5988);
#5078=AXIS2_PLACEMENT_3D('',#7354,#5990,#5991);
#5079=AXIS2_PLACEMENT_3D('',#7355,#5992,#5993);
#5080=AXIS2_PLACEMENT_3D('',#7356,#5994,#5995);
#5081=AXIS2_PLACEMENT_3D('',#7358,#5996,#5997);
#5082=AXIS2_PLACEMENT_3D('',#7361,#5999,#6000);
#5083=AXIS2_PLACEMENT_3D('',#7362,#6001,#6002);
#5084=AXIS2_PLACEMENT_3D('',#7364,#6003,#6004);
#5085=AXIS2_PLACEMENT_3D('',#7365,#6005,#6006);
#5086=AXIS2_PLACEMENT_3D('',#7367,#6007,#6008);
#5087=AXIS2_PLACEMENT_3D('',#7370,#6010,#6011);
#5088=AXIS2_PLACEMENT_3D('',#7371,#6012,#6013);
#5089=AXIS2_PLACEMENT_3D('',#7373,#6014,#6015);
#5090=AXIS2_PLACEMENT_3D('',#7374,#6016,#6017);
#5091=AXIS2_PLACEMENT_3D('',#7400,#6019,#6020);
#5092=AXIS2_PLACEMENT_3D('',#7419,#6021,#6022);
#5093=AXIS2_PLACEMENT_3D('',#7421,#6023,#6024);
#5094=AXIS2_PLACEMENT_3D('',#7424,#6026,#6027);
#5095=AXIS2_PLACEMENT_3D('',#7425,#6028,#6029);
#5096=AXIS2_PLACEMENT_3D('',#7426,#6030,#6031);
#5097=AXIS2_PLACEMENT_3D('',#7452,#6033,#6034);
#5098=AXIS2_PLACEMENT_3D('',#7471,#6035,#6036);
#5099=AXIS2_PLACEMENT_3D('',#7473,#6037,#6038);
#5100=AXIS2_PLACEMENT_3D('',#7476,#6040,#6041);
#5101=AXIS2_PLACEMENT_3D('',#7477,#6042,#6043);
#5102=AXIS2_PLACEMENT_3D('',#7478,#6044,#6045);
#5103=AXIS2_PLACEMENT_3D('',#7504,#6047,#6048);
#5104=AXIS2_PLACEMENT_3D('',#7523,#6049,#6050);
#5105=AXIS2_PLACEMENT_3D('',#7525,#6051,#6052);
#5106=AXIS2_PLACEMENT_3D('',#7528,#6054,#6055);
#5107=AXIS2_PLACEMENT_3D('',#7529,#6056,#6057);
#5108=AXIS2_PLACEMENT_3D('',#7530,#6058,#6059);
#5109=AXIS2_PLACEMENT_3D('',#7556,#6061,#6062);
#5110=AXIS2_PLACEMENT_3D('',#7575,#6063,#6064);
#5111=AXIS2_PLACEMENT_3D('',#7577,#6065,#6066);
#5112=AXIS2_PLACEMENT_3D('',#7580,#6068,#6069);
#5113=AXIS2_PLACEMENT_3D('',#7581,#6070,#6071);
#5114=AXIS2_PLACEMENT_3D('',#7582,#6072,#6073);
#5115=AXIS2_PLACEMENT_3D('',#7591,#6078,#6079);
#5116=AXIS2_PLACEMENT_3D('',#7597,#6082,#6083);
#5117=AXIS2_PLACEMENT_3D('',#7601,#6086,#6087);
#5118=AXIS2_PLACEMENT_3D('',#7605,#6090,#6091);
#5119=AXIS2_PLACEMENT_3D('',#7611,#6095,#6096);
#5120=AXIS2_PLACEMENT_3D('',#7615,#6099,#6100);
#5121=AXIS2_PLACEMENT_3D('',#7616,#6101,#6102);
#5122=AXIS2_PLACEMENT_3D('',#7618,#6104,#6105);
#5123=AXIS2_PLACEMENT_3D('',#7624,#6111,#6112);
#5124=AXIS2_PLACEMENT_3D('',#7633,#6117,#6118);
#5125=AXIS2_PLACEMENT_3D('',#7639,#6122,#6123);
#5126=AXIS2_PLACEMENT_3D('',#7645,#6127,#6128);
#5127=AXIS2_PLACEMENT_3D('',#7648,#6131,#6132);
#5128=AXIS2_PLACEMENT_3D('',#7649,#6133,#6134);
#5902=DIRECTION('axis',(0.,0.,1.));
#5903=DIRECTION('refdir',(1.,0.,0.));
#5904=DIRECTION('center_axis',(0.,1.,0.));
#5905=DIRECTION('ref_axis',(1.,0.,0.));
#5906=DIRECTION('center_axis',(0.,1.,0.));
#5907=DIRECTION('ref_axis',(1.,0.,0.));
#5908=DIRECTION('',(0.,1.,0.));
#5909=DIRECTION('center_axis',(0.,1.,0.));
#5910=DIRECTION('ref_axis',(1.,0.,0.));
#5911=DIRECTION('center_axis',(0.,1.,0.));
#5912=DIRECTION('ref_axis',(1.,0.,0.));
#5913=DIRECTION('center_axis',(0.,1.,0.));
#5914=DIRECTION('ref_axis',(1.,0.,0.));
#5915=DIRECTION('center_axis',(0.,1.,0.));
#5916=DIRECTION('ref_axis',(1.,0.,0.));
#5917=DIRECTION('',(0.,1.,0.));
#5918=DIRECTION('center_axis',(0.,1.,0.));
#5919=DIRECTION('ref_axis',(1.,0.,0.));
#5920=DIRECTION('center_axis',(0.,1.,0.));
#5921=DIRECTION('ref_axis',(1.,0.,0.));
#5922=DIRECTION('center_axis',(0.,0.,1.));
#5923=DIRECTION('ref_axis',(1.,0.,0.));
#5924=DIRECTION('center_axis',(0.,0.,1.));
#5925=DIRECTION('ref_axis',(1.,0.,0.));
#5926=DIRECTION('',(0.,0.,1.));
#5927=DIRECTION('center_axis',(0.,0.,1.));
#5928=DIRECTION('ref_axis',(1.,0.,0.));
#5929=DIRECTION('center_axis',(0.,0.,1.));
#5930=DIRECTION('ref_axis',(1.,0.,0.));
#5931=DIRECTION('center_axis',(0.,0.,1.));
#5932=DIRECTION('ref_axis',(1.,0.,0.));
#5933=DIRECTION('center_axis',(0.,0.,1.));
#5934=DIRECTION('ref_axis',(1.,0.,0.));
#5935=DIRECTION('',(0.,0.,1.));
#5936=DIRECTION('center_axis',(0.,0.,1.));
#5937=DIRECTION('ref_axis',(1.,0.,0.));
#5938=DIRECTION('center_axis',(0.,0.,1.));
#5939=DIRECTION('ref_axis',(1.,0.,0.));
#5940=DIRECTION('center_axis',(0.,0.,1.));
#5941=DIRECTION('ref_axis',(1.,0.,0.));
#5942=DIRECTION('center_axis',(0.,0.,1.));
#5943=DIRECTION('ref_axis',(1.,0.,0.));
#5944=DIRECTION('',(0.,0.,1.));
#5945=DIRECTION('center_axis',(0.,0.,1.));
#5946=DIRECTION('ref_axis',(1.,0.,0.));
#5947=DIRECTION('center_axis',(0.,0.,1.));
#5948=DIRECTION('ref_axis',(1.,0.,0.));
#5949=DIRECTION('center_axis',(0.,0.,1.));
#5950=DIRECTION('ref_axis',(1.,0.,0.));
#5951=DIRECTION('center_axis',(0.,0.,1.));
#5952=DIRECTION('ref_axis',(1.,0.,0.));
#5953=DIRECTION('',(0.,0.,1.));
#5954=DIRECTION('center_axis',(0.,0.,1.));
#5955=DIRECTION('ref_axis',(1.,0.,0.));
#5956=DIRECTION('center_axis',(0.,0.,1.));
#5957=DIRECTION('ref_axis',(1.,0.,0.));
#5958=DIRECTION('center_axis',(0.,0.,1.));
#5959=DIRECTION('ref_axis',(1.,0.,0.));
#5960=DIRECTION('center_axis',(0.,0.,1.));
#5961=DIRECTION('ref_axis',(1.,0.,0.));
#5962=DIRECTION('',(0.,0.,1.));
#5963=DIRECTION('center_axis',(0.,0.,1.));
#5964=DIRECTION('ref_axis',(1.,0.,0.));
#5965=DIRECTION('center_axis',(0.,0.,1.));
#5966=DIRECTION('ref_axis',(1.,0.,0.));
#5967=DIRECTION('center_axis',(0.,0.,1.));
#5968=DIRECTION('ref_axis',(1.,0.,0.));
#5969=DIRECTION('center_axis',(0.,0.,1.));
#5970=DIRECTION('ref_axis',(1.,0.,0.));
#5971=DIRECTION('',(0.,0.,1.));
#5972=DIRECTION('center_axis',(0.,0.,1.));
#5973=DIRECTION('ref_axis',(1.,0.,0.));
#5974=DIRECTION('center_axis',(0.,0.,1.));
#5975=DIRECTION('ref_axis',(1.,0.,0.));
#5976=DIRECTION('center_axis',(0.,0.,1.));
#5977=DIRECTION('ref_axis',(1.,0.,0.));
#5978=DIRECTION('center_axis',(0.,0.,1.));
#5979=DIRECTION('ref_axis',(1.,0.,0.));
#5980=DIRECTION('',(0.,0.,1.));
#5981=DIRECTION('center_axis',(0.,0.,1.));
#5982=DIRECTION('ref_axis',(1.,0.,0.));
#5983=DIRECTION('center_axis',(0.,0.,1.));
#5984=DIRECTION('ref_axis',(1.,0.,0.));
#5985=DIRECTION('center_axis',(0.,0.,1.));
#5986=DIRECTION('ref_axis',(1.,0.,0.));
#5987=DIRECTION('center_axis',(0.,0.,1.));
#5988=DIRECTION('ref_axis',(1.,0.,0.));
#5989=DIRECTION('',(0.,0.,1.));
#5990=DIRECTION('center_axis',(0.,0.,1.));
#5991=DIRECTION('ref_axis',(1.,0.,0.));
#5992=DIRECTION('center_axis',(0.,0.,1.));
#5993=DIRECTION('ref_axis',(1.,0.,0.));
#5994=DIRECTION('center_axis',(1.,0.,0.));
#5995=DIRECTION('ref_axis',(0.,0.,-1.));
#5996=DIRECTION('center_axis',(1.,0.,0.));
#5997=DIRECTION('ref_axis',(0.,0.,-1.));
#5998=DIRECTION('',(1.,0.,0.));
#5999=DIRECTION('center_axis',(-1.,0.,0.));
#6000=DIRECTION('ref_axis',(0.,0.,-1.));
#6001=DIRECTION('center_axis',(1.,0.,0.));
#6002=DIRECTION('ref_axis',(0.,0.,-1.));
#6003=DIRECTION('center_axis',(1.,0.,0.));
#6004=DIRECTION('ref_axis',(0.,0.,-1.));
#6005=DIRECTION('center_axis',(1.,0.,0.));
#6006=DIRECTION('ref_axis',(0.,0.,-1.));
#6007=DIRECTION('center_axis',(1.,0.,0.));
#6008=DIRECTION('ref_axis',(0.,0.,-1.));
#6009=DIRECTION('',(1.,0.,0.));
#6010=DIRECTION('center_axis',(1.,0.,0.));
#6011=DIRECTION('ref_axis',(0.,0.,-1.));
#6012=DIRECTION('center_axis',(1.,0.,0.));
#6013=DIRECTION('ref_axis',(0.,0.,-1.));
#6014=DIRECTION('center_axis',(-1.,0.,0.));
#6015=DIRECTION('ref_axis',(0.,0.,-1.));
#6016=DIRECTION('center_axis',(0.,0.,1.));
#6017=DIRECTION('ref_axis',(1.,0.,0.));
#6018=DIRECTION('',(0.,0.,1.));
#6019=DIRECTION('center_axis',(0.,0.,-1.));
#6020=DIRECTION('ref_axis',(1.,0.,0.));
#6021=DIRECTION('center_axis',(0.,0.,1.));
#6022=DIRECTION('ref_axis',(1.,0.,0.));
#6023=DIRECTION('center_axis',(0.,0.,1.));
#6024=DIRECTION('ref_axis',(1.,0.,0.));
#6025=DIRECTION('',(0.,0.,1.));
#6026=DIRECTION('center_axis',(0.,0.,-1.));
#6027=DIRECTION('ref_axis',(1.,0.,0.));
#6028=DIRECTION('center_axis',(0.,0.,1.));
#6029=DIRECTION('ref_axis',(1.,0.,0.));
#6030=DIRECTION('center_axis',(0.,0.,1.));
#6031=DIRECTION('ref_axis',(1.,0.,0.));
#6032=DIRECTION('',(0.,0.,1.));
#6033=DIRECTION('center_axis',(0.,0.,-1.));
#6034=DIRECTION('ref_axis',(1.,0.,0.));
#6035=DIRECTION('center_axis',(0.,0.,1.));
#6036=DIRECTION('ref_axis',(1.,0.,0.));
#6037=DIRECTION('center_axis',(0.,0.,1.));
#6038=DIRECTION('ref_axis',(1.,0.,0.));
#6039=DIRECTION('',(0.,0.,1.));
#6040=DIRECTION('center_axis',(0.,0.,-1.));
#6041=DIRECTION('ref_axis',(1.,0.,0.));
#6042=DIRECTION('center_axis',(0.,0.,1.));
#6043=DIRECTION('ref_axis',(1.,0.,0.));
#6044=DIRECTION('center_axis',(0.,0.,1.));
#6045=DIRECTION('ref_axis',(1.,0.,0.));
#6046=DIRECTION('',(0.,0.,1.));
#6047=DIRECTION('center_axis',(0.,0.,-1.));
#6048=DIRECTION('ref_axis',(1.,0.,0.));
#6049=DIRECTION('center_axis',(0.,0.,1.));
#6050=DIRECTION('ref_axis',(1.,0.,0.));
#6051=DIRECTION('center_axis',(0.,0.,1.));
#6052=DIRECTION('ref_axis',(1.,0.,0.));
#6053=DIRECTION('',(0.,0.,1.));
#6054=DIRECTION('center_axis',(0.,0.,-1.));
#6055=DIRECTION('ref_axis',(1.,0.,0.));
#6056=DIRECTION('center_axis',(0.,0.,1.));
#6057=DIRECTION('ref_axis',(1.,0.,0.));
#6058=DIRECTION('center_axis',(0.,0.,1.));
#6059=DIRECTION('ref_axis',(1.,0.,0.));
#6060=DIRECTION('',(0.,0.,1.));
#6061=DIRECTION('center_axis',(0.,0.,-1.));
#6062=DIRECTION('ref_axis',(1.,0.,0.));
#6063=DIRECTION('center_axis',(0.,0.,1.));
#6064=DIRECTION('ref_axis',(1.,0.,0.));
#6065=DIRECTION('center_axis',(0.,0.,1.));
#6066=DIRECTION('ref_axis',(1.,0.,0.));
#6067=DIRECTION('',(0.,0.,1.));
#6068=DIRECTION('center_axis',(0.,0.,-1.));
#6069=DIRECTION('ref_axis',(1.,0.,0.));
#6070=DIRECTION('center_axis',(0.,0.,1.));
#6071=DIRECTION('ref_axis',(1.,0.,0.));
#6072=DIRECTION('center_axis',(0.,-1.,0.));
#6073=DIRECTION('ref_axis',(1.,0.,0.));
#6074=DIRECTION('',(1.,0.,0.));
#6075=DIRECTION('',(0.,0.,1.));
#6076=DIRECTION('',(1.,0.,0.));
#6077=DIRECTION('',(0.,0.,1.));
#6078=DIRECTION('center_axis',(1.,0.,0.));
#6079=DIRECTION('ref_axis',(0.,1.,0.));
#6080=DIRECTION('',(0.,1.,0.));
#6081=DIRECTION('',(0.,1.,0.));
#6082=DIRECTION('center_axis',(-1.,0.,0.));
#6083=DIRECTION('ref_axis',(0.,0.,-1.));
#6084=DIRECTION('',(0.,1.,0.));
#6085=DIRECTION('',(0.,0.,1.));
#6086=DIRECTION('center_axis',(0.,0.,1.));
#6087=DIRECTION('ref_axis',(1.,0.,0.));
#6088=DIRECTION('',(-1.,0.,0.));
#6089=DIRECTION('',(0.,-1.,0.));
#6090=DIRECTION('center_axis',(0.,1.,0.));
#6091=DIRECTION('ref_axis',(-1.,0.,0.));
#6092=DIRECTION('',(-1.,0.,0.));
#6093=DIRECTION('',(-1.,0.,0.));
#6094=DIRECTION('',(0.,0.,1.));
#6095=DIRECTION('center_axis',(-1.,0.,0.));
#6096=DIRECTION('ref_axis',(0.,-1.,0.));
#6097=DIRECTION('',(0.,-1.,0.));
#6098=DIRECTION('',(0.,-1.,0.));
#6099=DIRECTION('center_axis',(1.,0.,0.));
#6100=DIRECTION('ref_axis',(0.,0.,-1.));
#6101=DIRECTION('center_axis',(0.,0.,1.));
#6102=DIRECTION('ref_axis',(1.,0.,0.));
#6103=DIRECTION('',(1.,0.,0.));
#6104=DIRECTION('center_axis',(1.,0.,0.));
#6105=DIRECTION('ref_axis',(0.,0.,-1.));
#6106=DIRECTION('',(1.,0.,0.));
#6107=DIRECTION('',(1.,0.,0.));
#6108=DIRECTION('',(1.,0.,0.));
#6109=DIRECTION('',(1.,0.,0.));
#6110=DIRECTION('',(1.,0.,0.));
#6111=DIRECTION('center_axis',(0.,1.,0.));
#6112=DIRECTION('ref_axis',(-1.,0.,0.));
#6113=DIRECTION('',(-1.,0.,0.));
#6114=DIRECTION('',(0.,0.,1.));
#6115=DIRECTION('',(-1.,0.,0.));
#6116=DIRECTION('',(0.,0.,1.));
#6117=DIRECTION('center_axis',(1.,0.,0.));
#6118=DIRECTION('ref_axis',(0.,1.,0.));
#6119=DIRECTION('',(0.,1.,0.));
#6120=DIRECTION('',(0.,1.,0.));
#6121=DIRECTION('',(0.,0.,1.));
#6122=DIRECTION('center_axis',(0.,-1.,0.));
#6123=DIRECTION('ref_axis',(1.,0.,0.));
#6124=DIRECTION('',(1.,0.,0.));
#6125=DIRECTION('',(1.,0.,0.));
#6126=DIRECTION('',(0.,0.,1.));
#6127=DIRECTION('center_axis',(-1.,0.,0.));
#6128=DIRECTION('ref_axis',(0.,-1.,0.));
#6129=DIRECTION('',(0.,-1.,0.));
#6130=DIRECTION('',(0.,-1.,0.));
#6131=DIRECTION('center_axis',(0.,0.,1.));
#6132=DIRECTION('ref_axis',(1.,0.,0.));
#6133=DIRECTION('center_axis',(0.,0.,1.));
#6134=DIRECTION('ref_axis',(1.,0.,0.));
#7285=CARTESIAN_POINT('',(0.,0.,0.));
#7286=CARTESIAN_POINT('Origin',(-4.5,-1.8,4.));
#7287=CARTESIAN_POINT('',(-4.665,-1.75,4.));
#7288=CARTESIAN_POINT('Origin',(-4.5,-1.75,4.));
#7289=CARTESIAN_POINT('',(-4.665,-0.8,4.));
#7290=CARTESIAN_POINT('',(-4.665,-1.8,4.));
#7291=CARTESIAN_POINT('Origin',(-4.5,-0.8,4.));
#7292=CARTESIAN_POINT('Origin',(-4.5,-0.8,4.));
#7293=CARTESIAN_POINT('Origin',(4.5,-1.8,4.));
#7294=CARTESIAN_POINT('',(4.335,-1.75,4.));
#7295=CARTESIAN_POINT('Origin',(4.5,-1.75,4.));
#7296=CARTESIAN_POINT('',(4.335,-0.8,4.));
#7297=CARTESIAN_POINT('',(4.335,-1.8,4.));
#7298=CARTESIAN_POINT('Origin',(4.5,-0.8,4.));
#7299=CARTESIAN_POINT('Origin',(4.5,-0.8,4.));
#7300=CARTESIAN_POINT('Origin',(5.,0.,1.3));
#7301=CARTESIAN_POINT('',(4.85,-1.83697019872103E-17,2.));
#7302=CARTESIAN_POINT('Origin',(5.,0.,2.));
#7303=CARTESIAN_POINT('',(4.85,-1.83697019872103E-17,2.4));
#7304=CARTESIAN_POINT('',(4.85,-1.83697019872103E-17,1.3));
#7305=CARTESIAN_POINT('Origin',(5.,0.,2.4));
#7306=CARTESIAN_POINT('Origin',(5.,0.,2.4));
#7307=CARTESIAN_POINT('Origin',(-5.,0.,1.3));
#7308=CARTESIAN_POINT('',(-5.15,-1.83697019872103E-17,2.));
#7309=CARTESIAN_POINT('Origin',(-5.,0.,2.));
#7310=CARTESIAN_POINT('',(-5.15,-1.83697019872103E-17,2.4));
#7311=CARTESIAN_POINT('',(-5.15,-1.83697019872103E-17,1.3));
#7312=CARTESIAN_POINT('Origin',(-5.,0.,2.4));
#7313=CARTESIAN_POINT('Origin',(-5.,0.,2.4));
#7314=CARTESIAN_POINT('Origin',(4.5,-1.4,1.9));
#7315=CARTESIAN_POINT('',(4.335,-1.4,2.));
#7316=CARTESIAN_POINT('Origin',(4.5,-1.4,2.));
#7317=CARTESIAN_POINT('',(4.335,-1.4,3.2));
#7318=CARTESIAN_POINT('',(4.335,-1.4,1.9));
#7319=CARTESIAN_POINT('Origin',(4.5,-1.4,3.2));
#7320=CARTESIAN_POINT('Origin',(4.5,-1.4,3.2));
#7321=CARTESIAN_POINT('Origin',(-4.5,-1.4,1.9));
#7322=CARTESIAN_POINT('',(-4.665,-1.4,2.));
#7323=CARTESIAN_POINT('Origin',(-4.5,-1.4,2.));
#7324=CARTESIAN_POINT('',(-4.665,-1.4,3.2));
#7325=CARTESIAN_POINT('',(-4.665,-1.4,1.9));
#7326=CARTESIAN_POINT('Origin',(-4.5,-1.4,3.2));
#7327=CARTESIAN_POINT('Origin',(-4.5,-1.4,3.2));
#7328=CARTESIAN_POINT('Origin',(-4.5,1.4,1.9));
#7329=CARTESIAN_POINT('',(-4.665,1.4,2.));
#7330=CARTESIAN_POINT('Origin',(-4.5,1.4,2.));
#7331=CARTESIAN_POINT('',(-4.665,1.4,3.2));
#7332=CARTESIAN_POINT('',(-4.665,1.4,1.9));
#7333=CARTESIAN_POINT('Origin',(-4.5,1.4,3.2));
#7334=CARTESIAN_POINT('Origin',(-4.5,1.4,3.2));
#7335=CARTESIAN_POINT('Origin',(0.,-1.4,1.9));
#7336=CARTESIAN_POINT('',(-0.165,-1.4,2.));
#7337=CARTESIAN_POINT('Origin',(0.,-1.4,2.));
#7338=CARTESIAN_POINT('',(-0.165,-1.4,3.2));
#7339=CARTESIAN_POINT('',(-0.165,-1.4,1.9));
#7340=CARTESIAN_POINT('Origin',(0.,-1.4,3.2));
#7341=CARTESIAN_POINT('Origin',(0.,-1.4,3.2));
#7342=CARTESIAN_POINT('Origin',(0.,1.4,1.9));
#7343=CARTESIAN_POINT('',(-0.165,1.4,2.));
#7344=CARTESIAN_POINT('Origin',(0.,1.4,2.));
#7345=CARTESIAN_POINT('',(-0.165,1.4,3.2));
#7346=CARTESIAN_POINT('',(-0.165,1.4,1.9));
#7347=CARTESIAN_POINT('Origin',(0.,1.4,3.2));
#7348=CARTESIAN_POINT('Origin',(0.,1.4,3.2));
#7349=CARTESIAN_POINT('Origin',(4.5,1.4,1.9));
#7350=CARTESIAN_POINT('',(4.335,1.4,2.));
#7351=CARTESIAN_POINT('Origin',(4.5,1.4,2.));
#7352=CARTESIAN_POINT('',(4.335,1.4,3.2));
#7353=CARTESIAN_POINT('',(4.335,1.4,1.9));
#7354=CARTESIAN_POINT('Origin',(4.5,1.4,3.2));
#7355=CARTESIAN_POINT('Origin',(4.5,1.4,3.2));
#7356=CARTESIAN_POINT('Origin',(4.1,0.,3.5));
#7357=CARTESIAN_POINT('',(4.1,-8.38883057415937E-17,4.185));
#7358=CARTESIAN_POINT('Origin',(4.1,0.,3.5));
#7359=CARTESIAN_POINT('',(5.5,8.38883057415937E-17,4.185));
#7360=CARTESIAN_POINT('',(4.1,-8.38883057415937E-17,4.185));
#7361=CARTESIAN_POINT('Origin',(5.5,0.,3.5));
#7362=CARTESIAN_POINT('Origin',(4.1,0.,3.5));
#7363=CARTESIAN_POINT('',(4.1,-3.67394039744206E-17,3.8));
#7364=CARTESIAN_POINT('Origin',(4.1,0.,3.5));
#7365=CARTESIAN_POINT('Origin',(-5.6,0.,3.5));
#7366=CARTESIAN_POINT('',(-5.5,-8.38883057415937E-17,4.185));
#7367=CARTESIAN_POINT('Origin',(-5.5,0.,3.5));
#7368=CARTESIAN_POINT('',(-4.1,-8.38883057415937E-17,4.185));
#7369=CARTESIAN_POINT('',(-5.6,-8.38883057415937E-17,4.185));
#7370=CARTESIAN_POINT('Origin',(-4.1,0.,3.5));
#7371=CARTESIAN_POINT('Origin',(-4.1,0.,3.5));
#7372=CARTESIAN_POINT('',(-4.1,3.67394039744206E-17,3.8));
#7373=CARTESIAN_POINT('Origin',(-4.1,0.,3.5));
#7374=CARTESIAN_POINT('Origin',(3.75,0.,3.4));
#7375=CARTESIAN_POINT('',(3.75,-0.2,3.72360679774998));
#7376=CARTESIAN_POINT('',(3.95,1.4590044056349E-17,3.8));
#7377=CARTESIAN_POINT('Ctrl Pts',(3.75,-0.2,3.72360679774998));
#7378=CARTESIAN_POINT('Ctrl Pts',(3.77630182346442,-0.2,3.72360679774998));
#7379=CARTESIAN_POINT('Ctrl Pts',(3.80333179602069,-0.194568877616075,3.72872056892082));
#7380=CARTESIAN_POINT('Ctrl Pts',(3.85213335089966,-0.173983137835284,3.74474475389314));
#7381=CARTESIAN_POINT('Ctrl Pts',(3.87402433525872,-0.158818377215904,3.75527603224183));
#7382=CARTESIAN_POINT('Ctrl Pts',(3.90862698590243,-0.124215726572194,3.77377192701083));
#7383=CARTESIAN_POINT('Ctrl Pts',(3.92391823287771,-0.102283014436697,3.78316729552365));
#7384=CARTESIAN_POINT('Ctrl Pts',(3.94462445314031,-0.0532042473651336,
3.79633569102376));
#7385=CARTESIAN_POINT('Ctrl Pts',(3.95,-0.0260124669966692,3.8));
#7386=CARTESIAN_POINT('Ctrl Pts',(3.95,9.71445146547012E-17,3.8));
#7387=CARTESIAN_POINT('',(3.55,-2.43895323233112E-17,3.8));
#7388=CARTESIAN_POINT('Ctrl Pts',(3.55,-2.77555756156289E-17,3.8));
#7389=CARTESIAN_POINT('Ctrl Pts',(3.55,-0.0260124669966693,3.8));
#7390=CARTESIAN_POINT('Ctrl Pts',(3.55537554685969,-0.0532042473651339,
3.79633569102376));
#7391=CARTESIAN_POINT('Ctrl Pts',(3.57608176712229,-0.102283014436697,3.78316729552365));
#7392=CARTESIAN_POINT('Ctrl Pts',(3.59137301409757,-0.124215726572194,3.77377192701083));
#7393=CARTESIAN_POINT('Ctrl Pts',(3.62597566474128,-0.158818377215904,3.75527603224183));
#7394=CARTESIAN_POINT('Ctrl Pts',(3.64786664910034,-0.173983137835283,3.74474475389314));
#7395=CARTESIAN_POINT('Ctrl Pts',(3.69666820397931,-0.194568877616075,3.72872056892082));
#7396=CARTESIAN_POINT('Ctrl Pts',(3.72369817653558,-0.2,3.72360679774998));
#7397=CARTESIAN_POINT('Ctrl Pts',(3.75,-0.2,3.72360679774998));
#7398=CARTESIAN_POINT('',(3.55,2.44929359829471E-17,4.35));
#7399=CARTESIAN_POINT('',(3.55,-2.44929359829471E-17,3.4));
#7400=CARTESIAN_POINT('Origin',(3.75,0.,4.35));
#7401=CARTESIAN_POINT('Ctrl Pts',(3.95,6.24500451351651E-17,3.8));
#7402=CARTESIAN_POINT('Ctrl Pts',(3.95,0.0260124669966693,3.8));
#7403=CARTESIAN_POINT('Ctrl Pts',(3.94462445314031,0.0532042473651336,3.79633569102376));
#7404=CARTESIAN_POINT('Ctrl Pts',(3.92391823287771,0.102283014436697,3.78316729552365));
#7405=CARTESIAN_POINT('Ctrl Pts',(3.90862698590243,0.124215726572194,3.77377192701083));
#7406=CARTESIAN_POINT('Ctrl Pts',(3.87402433525872,0.158818377215904,3.75527603224183));
#7407=CARTESIAN_POINT('Ctrl Pts',(3.85213335089966,0.173983137835284,3.74474475389314));
#7408=CARTESIAN_POINT('Ctrl Pts',(3.80333179602069,0.194568877616075,3.72872056892082));
#7409=CARTESIAN_POINT('Ctrl Pts',(3.77630182346442,0.2,3.72360679774998));
#7410=CARTESIAN_POINT('Ctrl Pts',(3.72369817653558,0.2,3.72360679774998));
#7411=CARTESIAN_POINT('Ctrl Pts',(3.69666820397931,0.194568877616075,3.72872056892082));
#7412=CARTESIAN_POINT('Ctrl Pts',(3.64786664910035,0.173983137835284,3.74474475389314));
#7413=CARTESIAN_POINT('Ctrl Pts',(3.62597566474128,0.158818377215904,3.75527603224183));
#7414=CARTESIAN_POINT('Ctrl Pts',(3.59137301409757,0.124215726572194,3.77377192701083));
#7415=CARTESIAN_POINT('Ctrl Pts',(3.57608176712229,0.102283014436697,3.78316729552365));
#7416=CARTESIAN_POINT('Ctrl Pts',(3.55537554685969,0.0532042473651339,3.79633569102376));
#7417=CARTESIAN_POINT('Ctrl Pts',(3.55,0.0260124669966693,3.8));
#7418=CARTESIAN_POINT('Ctrl Pts',(3.55,-2.77555756156289E-17,3.8));
#7419=CARTESIAN_POINT('Origin',(3.75,0.,4.35));
#7420=CARTESIAN_POINT('',(3.235,-6.30693101560886E-17,4.35));
#7421=CARTESIAN_POINT('Origin',(3.75,0.,4.35));
#7422=CARTESIAN_POINT('',(3.235,6.30693101560886E-17,5.));
#7423=CARTESIAN_POINT('',(3.235,-6.30693101560886E-17,4.35));
#7424=CARTESIAN_POINT('Origin',(3.75,0.,5.));
#7425=CARTESIAN_POINT('Origin',(3.75,0.,4.35));
#7426=CARTESIAN_POINT('Origin',(1.25,0.,3.4));
#7427=CARTESIAN_POINT('',(1.25,-0.2,3.72360679774998));
#7428=CARTESIAN_POINT('',(1.45,-1.02246722744222E-18,3.8));
#7429=CARTESIAN_POINT('Ctrl Pts',(1.25,-0.2,3.72360679774998));
#7430=CARTESIAN_POINT('Ctrl Pts',(1.27630182346442,-0.2,3.72360679774998));
#7431=CARTESIAN_POINT('Ctrl Pts',(1.30333179602069,-0.194568877616075,3.72872056892082));
#7432=CARTESIAN_POINT('Ctrl Pts',(1.35213335089965,-0.173983137835284,3.74474475389314));
#7433=CARTESIAN_POINT('Ctrl Pts',(1.37402433525871,-0.158818377215904,3.75527603224183));
#7434=CARTESIAN_POINT('Ctrl Pts',(1.40862698590242,-0.124215726572194,3.77377192701083));
#7435=CARTESIAN_POINT('Ctrl Pts',(1.42391823287771,-0.102283014436697,3.78316729552365));
#7436=CARTESIAN_POINT('Ctrl Pts',(1.44462445314031,-0.0532042473651338,
3.79633569102376));
#7437=CARTESIAN_POINT('Ctrl Pts',(1.45,-0.0260124669966693,3.8));
#7438=CARTESIAN_POINT('Ctrl Pts',(1.45,3.46944695195361E-17,3.8));
#7439=CARTESIAN_POINT('',(1.05,-2.6124255799288E-17,3.8));
#7440=CARTESIAN_POINT('Ctrl Pts',(1.05,-2.08166817117217E-17,3.8));
#7441=CARTESIAN_POINT('Ctrl Pts',(1.05,-0.0260124669966693,3.8));
#7442=CARTESIAN_POINT('Ctrl Pts',(1.05537554685969,-0.0532042473651339,
3.79633569102376));
#7443=CARTESIAN_POINT('Ctrl Pts',(1.07608176712229,-0.102283014436697,3.78316729552365));
#7444=CARTESIAN_POINT('Ctrl Pts',(1.09137301409758,-0.124215726572194,3.77377192701083));
#7445=CARTESIAN_POINT('Ctrl Pts',(1.12597566474129,-0.158818377215904,3.75527603224183));
#7446=CARTESIAN_POINT('Ctrl Pts',(1.14786664910035,-0.173983137835284,3.74474475389314));
#7447=CARTESIAN_POINT('Ctrl Pts',(1.19666820397931,-0.194568877616075,3.72872056892082));
#7448=CARTESIAN_POINT('Ctrl Pts',(1.22369817653558,-0.2,3.72360679774998));
#7449=CARTESIAN_POINT('Ctrl Pts',(1.25,-0.2,3.72360679774998));
#7450=CARTESIAN_POINT('',(1.05,2.44929359829471E-17,4.35));
#7451=CARTESIAN_POINT('',(1.05,-2.44929359829471E-17,3.4));
#7452=CARTESIAN_POINT('Origin',(1.25,0.,4.35));
#7453=CARTESIAN_POINT('Ctrl Pts',(1.45,2.77555756156289E-17,3.8));
#7454=CARTESIAN_POINT('Ctrl Pts',(1.45,0.0260124669966693,3.8));
#7455=CARTESIAN_POINT('Ctrl Pts',(1.44462445314031,0.0532042473651337,3.79633569102376));
#7456=CARTESIAN_POINT('Ctrl Pts',(1.42391823287771,0.102283014436697,3.78316729552365));
#7457=CARTESIAN_POINT('Ctrl Pts',(1.40862698590243,0.124215726572194,3.77377192701083));
#7458=CARTESIAN_POINT('Ctrl Pts',(1.37402433525872,0.158818377215904,3.75527603224183));
#7459=CARTESIAN_POINT('Ctrl Pts',(1.35213335089966,0.173983137835283,3.74474475389314));
#7460=CARTESIAN_POINT('Ctrl Pts',(1.30333179602069,0.194568877616075,3.72872056892082));
#7461=CARTESIAN_POINT('Ctrl Pts',(1.27630182346442,0.2,3.72360679774998));
#7462=CARTESIAN_POINT('Ctrl Pts',(1.22369817653558,0.2,3.72360679774998));
#7463=CARTESIAN_POINT('Ctrl Pts',(1.19666820397931,0.194568877616075,3.72872056892082));
#7464=CARTESIAN_POINT('Ctrl Pts',(1.14786664910035,0.173983137835284,3.74474475389314));
#7465=CARTESIAN_POINT('Ctrl Pts',(1.12597566474129,0.158818377215904,3.75527603224183));
#7466=CARTESIAN_POINT('Ctrl Pts',(1.09137301409758,0.124215726572194,3.77377192701083));
#7467=CARTESIAN_POINT('Ctrl Pts',(1.07608176712229,0.102283014436697,3.78316729552365));
#7468=CARTESIAN_POINT('Ctrl Pts',(1.05537554685969,0.0532042473651338,3.79633569102376));
#7469=CARTESIAN_POINT('Ctrl Pts',(1.05,0.0260124669966694,3.8));
#7470=CARTESIAN_POINT('Ctrl Pts',(1.05,4.16333634234434E-17,3.8));
#7471=CARTESIAN_POINT('Origin',(1.25,0.,4.35));
#7472=CARTESIAN_POINT('',(0.735,-6.30693101560887E-17,4.35));
#7473=CARTESIAN_POINT('Origin',(1.25,0.,4.35));
#7474=CARTESIAN_POINT('',(0.735,6.30693101560887E-17,5.));
#7475=CARTESIAN_POINT('',(0.735,-6.30693101560887E-17,4.35));
#7476=CARTESIAN_POINT('Origin',(1.25,0.,5.));
#7477=CARTESIAN_POINT('Origin',(1.25,0.,4.35));
#7478=CARTESIAN_POINT('Origin',(-1.25,0.,3.4));
#7479=CARTESIAN_POINT('',(-1.25,-0.2,3.72360679774998));
#7480=CARTESIAN_POINT('',(-1.05,-2.53085958911175E-17,3.8));
#7481=CARTESIAN_POINT('Ctrl Pts',(-1.25,-0.2,3.72360679774998));
#7482=CARTESIAN_POINT('Ctrl Pts',(-1.22369817653558,-0.2,3.72360679774998));
#7483=CARTESIAN_POINT('Ctrl Pts',(-1.19666820397931,-0.194568877616075,
3.72872056892082));
#7484=CARTESIAN_POINT('Ctrl Pts',(-1.14786664910035,-0.173983137835284,
3.74474475389314));
#7485=CARTESIAN_POINT('Ctrl Pts',(-1.12597566474129,-0.158818377215904,
3.75527603224183));
#7486=CARTESIAN_POINT('Ctrl Pts',(-1.09137301409758,-0.124215726572194,
3.77377192701083));
#7487=CARTESIAN_POINT('Ctrl Pts',(-1.07608176712229,-0.102283014436697,
3.78316729552365));
#7488=CARTESIAN_POINT('Ctrl Pts',(-1.05537554685969,-0.0532042473651338,
3.79633569102376));
#7489=CARTESIAN_POINT('Ctrl Pts',(-1.05,-0.0260124669966693,3.8));
#7490=CARTESIAN_POINT('Ctrl Pts',(-1.05,5.55111512312578E-17,3.8));
#7491=CARTESIAN_POINT('',(-1.45,-1.91853618953807E-17,3.8));
#7492=CARTESIAN_POINT('Ctrl Pts',(-1.45,-2.77555756156289E-17,3.8));
#7493=CARTESIAN_POINT('Ctrl Pts',(-1.45,-0.0260124669966693,3.8));
#7494=CARTESIAN_POINT('Ctrl Pts',(-1.44462445314031,-0.0532042473651339,
3.79633569102376));
#7495=CARTESIAN_POINT('Ctrl Pts',(-1.42391823287771,-0.102283014436697,
3.78316729552365));
#7496=CARTESIAN_POINT('Ctrl Pts',(-1.40862698590242,-0.124215726572194,
3.77377192701083));
#7497=CARTESIAN_POINT('Ctrl Pts',(-1.37402433525871,-0.158818377215904,
3.75527603224183));
#7498=CARTESIAN_POINT('Ctrl Pts',(-1.35213335089965,-0.173983137835284,
3.74474475389314));
#7499=CARTESIAN_POINT('Ctrl Pts',(-1.30333179602069,-0.194568877616075,
3.72872056892082));
#7500=CARTESIAN_POINT('Ctrl Pts',(-1.27630182346442,-0.2,3.72360679774998));
#7501=CARTESIAN_POINT('Ctrl Pts',(-1.25,-0.2,3.72360679774998));
#7502=CARTESIAN_POINT('',(-1.45,2.44929359829471E-17,4.35));
#7503=CARTESIAN_POINT('',(-1.45,-2.44929359829471E-17,3.4));
#7504=CARTESIAN_POINT('Origin',(-1.25,0.,4.35));
#7505=CARTESIAN_POINT('Ctrl Pts',(-1.05,-1.38777878078145E-17,3.8));
#7506=CARTESIAN_POINT('Ctrl Pts',(-1.05,0.0260124669966692,3.8));
#7507=CARTESIAN_POINT('Ctrl Pts',(-1.05537554685969,0.0532042473651337,
3.79633569102376));
#7508=CARTESIAN_POINT('Ctrl Pts',(-1.07608176712229,0.102283014436697,3.78316729552365));
#7509=CARTESIAN_POINT('Ctrl Pts',(-1.09137301409757,0.124215726572194,3.77377192701083));
#7510=CARTESIAN_POINT('Ctrl Pts',(-1.12597566474128,0.158818377215904,3.75527603224183));
#7511=CARTESIAN_POINT('Ctrl Pts',(-1.14786664910034,0.173983137835283,3.74474475389314));
#7512=CARTESIAN_POINT('Ctrl Pts',(-1.19666820397931,0.194568877616075,3.72872056892082));
#7513=CARTESIAN_POINT('Ctrl Pts',(-1.22369817653558,0.2,3.72360679774998));
#7514=CARTESIAN_POINT('Ctrl Pts',(-1.27630182346442,0.2,3.72360679774998));
#7515=CARTESIAN_POINT('Ctrl Pts',(-1.30333179602069,0.194568877616075,3.72872056892082));
#7516=CARTESIAN_POINT('Ctrl Pts',(-1.35213335089965,0.173983137835284,3.74474475389314));
#7517=CARTESIAN_POINT('Ctrl Pts',(-1.37402433525871,0.158818377215904,3.75527603224183));
#7518=CARTESIAN_POINT('Ctrl Pts',(-1.40862698590242,0.124215726572194,3.77377192701083));
#7519=CARTESIAN_POINT('Ctrl Pts',(-1.42391823287771,0.102283014436697,3.78316729552365));
#7520=CARTESIAN_POINT('Ctrl Pts',(-1.44462445314031,0.0532042473651338,
3.79633569102376));
#7521=CARTESIAN_POINT('Ctrl Pts',(-1.45,0.0260124669966693,3.8));
#7522=CARTESIAN_POINT('Ctrl Pts',(-1.45,-3.81639164714898E-17,3.8));
#7523=CARTESIAN_POINT('Origin',(-1.25,0.,4.35));
#7524=CARTESIAN_POINT('',(-1.765,-6.30693101560887E-17,4.35));
#7525=CARTESIAN_POINT('Origin',(-1.25,0.,4.35));
#7526=CARTESIAN_POINT('',(-1.765,6.30693101560887E-17,5.));
#7527=CARTESIAN_POINT('',(-1.765,-6.30693101560887E-17,4.35));
#7528=CARTESIAN_POINT('Origin',(-1.25,0.,5.));
#7529=CARTESIAN_POINT('Origin',(-1.25,0.,4.35));
#7530=CARTESIAN_POINT('Origin',(-3.75,0.,3.4));
#7531=CARTESIAN_POINT('',(-3.75,-0.2,3.72360679774998));
#7532=CARTESIAN_POINT('',(-3.55,4.1817032004882E-18,3.8));
#7533=CARTESIAN_POINT('Ctrl Pts',(-3.75,-0.2,3.72360679774998));
#7534=CARTESIAN_POINT('Ctrl Pts',(-3.72369817653558,-0.2,3.72360679774998));
#7535=CARTESIAN_POINT('Ctrl Pts',(-3.69666820397931,-0.194568877616075,
3.72872056892082));
#7536=CARTESIAN_POINT('Ctrl Pts',(-3.64786664910034,-0.173983137835284,
3.74474475389314));
#7537=CARTESIAN_POINT('Ctrl Pts',(-3.62597566474128,-0.158818377215904,
3.75527603224183));
#7538=CARTESIAN_POINT('Ctrl Pts',(-3.59137301409757,-0.124215726572194,
3.77377192701083));
#7539=CARTESIAN_POINT('Ctrl Pts',(-3.57608176712229,-0.102283014436697,
3.78316729552365));
#7540=CARTESIAN_POINT('Ctrl Pts',(-3.55537554685969,-0.0532042473651337,
3.79633569102376));
#7541=CARTESIAN_POINT('Ctrl Pts',(-3.55,-0.0260124669966693,3.8));
#7542=CARTESIAN_POINT('Ctrl Pts',(-3.55,6.24500451351651E-17,3.8));
#7543=CARTESIAN_POINT('',(-3.95,-2.09200853713576E-17,3.8));
#7544=CARTESIAN_POINT('Ctrl Pts',(-3.95,-1.73472347597681E-17,3.8));
#7545=CARTESIAN_POINT('Ctrl Pts',(-3.95,-0.0260124669966693,3.8));
#7546=CARTESIAN_POINT('Ctrl Pts',(-3.94462445314031,-0.0532042473651343,
3.79633569102376));
#7547=CARTESIAN_POINT('Ctrl Pts',(-3.92391823287771,-0.102283014436697,
3.78316729552365));
#7548=CARTESIAN_POINT('Ctrl Pts',(-3.90862698590243,-0.124215726572194,
3.77377192701083));
#7549=CARTESIAN_POINT('Ctrl Pts',(-3.87402433525872,-0.158818377215904,
3.75527603224183));
#7550=CARTESIAN_POINT('Ctrl Pts',(-3.85213335089965,-0.173983137835284,
3.74474475389314));
#7551=CARTESIAN_POINT('Ctrl Pts',(-3.80333179602069,-0.194568877616075,
3.72872056892082));
#7552=CARTESIAN_POINT('Ctrl Pts',(-3.77630182346442,-0.2,3.72360679774998));
#7553=CARTESIAN_POINT('Ctrl Pts',(-3.75,-0.2,3.72360679774998));
#7554=CARTESIAN_POINT('',(-3.95,2.44929359829471E-17,4.35));
#7555=CARTESIAN_POINT('',(-3.95,-2.44929359829471E-17,3.4));
#7556=CARTESIAN_POINT('Origin',(-3.75,0.,4.35));
#7557=CARTESIAN_POINT('Ctrl Pts',(-3.55,3.81639164714898E-17,3.8));
#7558=CARTESIAN_POINT('Ctrl Pts',(-3.55,0.0260124669966693,3.8));
#7559=CARTESIAN_POINT('Ctrl Pts',(-3.55537554685969,0.0532042473651338,
3.79633569102376));
#7560=CARTESIAN_POINT('Ctrl Pts',(-3.57608176712229,0.102283014436697,3.78316729552365));
#7561=CARTESIAN_POINT('Ctrl Pts',(-3.59137301409758,0.124215726572194,3.77377192701083));
#7562=CARTESIAN_POINT('Ctrl Pts',(-3.62597566474129,0.158818377215904,3.75527603224183));
#7563=CARTESIAN_POINT('Ctrl Pts',(-3.64786664910034,0.173983137835284,3.74474475389314));
#7564=CARTESIAN_POINT('Ctrl Pts',(-3.69666820397931,0.194568877616075,3.72872056892082));
#7565=CARTESIAN_POINT('Ctrl Pts',(-3.72369817653558,0.2,3.72360679774998));
#7566=CARTESIAN_POINT('Ctrl Pts',(-3.77630182346442,0.2,3.72360679774998));
#7567=CARTESIAN_POINT('Ctrl Pts',(-3.80333179602069,0.194568877616075,3.72872056892082));
#7568=CARTESIAN_POINT('Ctrl Pts',(-3.85213335089965,0.173983137835284,3.74474475389314));
#7569=CARTESIAN_POINT('Ctrl Pts',(-3.87402433525872,0.158818377215904,3.75527603224183));
#7570=CARTESIAN_POINT('Ctrl Pts',(-3.90862698590243,0.124215726572194,3.77377192701083));
#7571=CARTESIAN_POINT('Ctrl Pts',(-3.92391823287771,0.102283014436697,3.78316729552365));
#7572=CARTESIAN_POINT('Ctrl Pts',(-3.94462445314031,0.0532042473651338,
3.79633569102376));
#7573=CARTESIAN_POINT('Ctrl Pts',(-3.95,0.0260124669966692,3.8));
#7574=CARTESIAN_POINT('Ctrl Pts',(-3.95,-1.17961196366423E-16,3.8));
#7575=CARTESIAN_POINT('Origin',(-3.75,0.,4.35));
#7576=CARTESIAN_POINT('',(-4.265,-6.30693101560887E-17,4.35));
#7577=CARTESIAN_POINT('Origin',(-3.75,0.,4.35));
#7578=CARTESIAN_POINT('',(-4.265,6.30693101560887E-17,5.));
#7579=CARTESIAN_POINT('',(-4.265,-6.30693101560887E-17,4.35));
#7580=CARTESIAN_POINT('Origin',(-3.75,0.,5.));
#7581=CARTESIAN_POINT('Origin',(-3.75,0.,4.35));
#7582=CARTESIAN_POINT('Origin',(-4.,-0.8,1.9));
#7583=CARTESIAN_POINT('',(-4.,-0.8,2.));
#7584=CARTESIAN_POINT('',(4.,-0.8,2.));
#7585=CARTESIAN_POINT('',(-2.,-0.8,2.));
#7586=CARTESIAN_POINT('',(-4.,-0.8,3.5));
#7587=CARTESIAN_POINT('',(-4.,-0.8,1.9));
#7588=CARTESIAN_POINT('',(4.,-0.8,3.5));
#7589=CARTESIAN_POINT('',(-4.,-0.8,3.5));
#7590=CARTESIAN_POINT('',(4.,-0.8,1.9));
#7591=CARTESIAN_POINT('Origin',(4.,-0.8,1.9));
#7592=CARTESIAN_POINT('',(4.,0.8,2.));
#7593=CARTESIAN_POINT('',(4.,-0.4,2.));
#7594=CARTESIAN_POINT('',(4.,-0.3,3.5));
#7595=CARTESIAN_POINT('',(4.,-0.8,3.5));
#7596=CARTESIAN_POINT('',(4.,0.3,3.5));
#7597=CARTESIAN_POINT('Origin',(4.,0.,3.5));
#7598=CARTESIAN_POINT('',(4.,0.8,3.5));
#7599=CARTESIAN_POINT('',(4.,-0.8,3.5));
#7600=CARTESIAN_POINT('',(4.,0.8,1.9));
#7601=CARTESIAN_POINT('Origin',(0.,0.,3.5));
#7602=CARTESIAN_POINT('',(-4.,-0.3,3.5));
#7603=CARTESIAN_POINT('',(-5.6,-0.3,3.5));
#7604=CARTESIAN_POINT('',(-4.,0.8,3.5));
#7605=CARTESIAN_POINT('Origin',(4.,0.8,1.9));
#7606=CARTESIAN_POINT('',(-4.,0.8,2.));
#7607=CARTESIAN_POINT('',(2.,0.8,2.));
#7608=CARTESIAN_POINT('',(-4.,0.8,3.5));
#7609=CARTESIAN_POINT('',(4.,0.8,3.5));
#7610=CARTESIAN_POINT('',(-4.,0.8,1.9));
#7611=CARTESIAN_POINT('Origin',(-4.,0.8,1.9));
#7612=CARTESIAN_POINT('',(-4.,0.4,2.));
#7613=CARTESIAN_POINT('',(-4.,0.3,3.5));
#7614=CARTESIAN_POINT('',(-4.,0.8,3.5));
#7615=CARTESIAN_POINT('Origin',(-4.,0.,3.5));
#7616=CARTESIAN_POINT('Origin',(0.,0.,3.5));
#7617=CARTESIAN_POINT('',(-5.6,0.3,3.5));
#7618=CARTESIAN_POINT('Origin',(-5.6,0.,3.5));
#7619=CARTESIAN_POINT('',(-5.6,-3.67394039744206E-17,3.8));
#7620=CARTESIAN_POINT('',(-5.6,-3.67394039744206E-17,3.8));
#7621=CARTESIAN_POINT('',(-5.6,-3.67394039744206E-17,3.8));
#7622=CARTESIAN_POINT('',(-5.6,-3.67394039744206E-17,3.8));
#7623=CARTESIAN_POINT('',(-5.6,-3.67394039744206E-17,3.8));
#7624=CARTESIAN_POINT('Origin',(5.5,1.75,2.));
#7625=CARTESIAN_POINT('',(5.5,1.75,2.));
#7626=CARTESIAN_POINT('',(-5.5,1.75,2.));
#7627=CARTESIAN_POINT('',(5.5,1.75,2.));
#7628=CARTESIAN_POINT('',(-5.5,1.75,5.));
#7629=CARTESIAN_POINT('',(-5.5,1.75,2.));
#7630=CARTESIAN_POINT('',(5.5,1.75,5.));
#7631=CARTESIAN_POINT('',(5.5,1.75,5.));
#7632=CARTESIAN_POINT('',(5.5,1.75,2.));
#7633=CARTESIAN_POINT('Origin',(5.5,-1.75,2.));
#7634=CARTESIAN_POINT('',(5.5,-1.75,2.));
#7635=CARTESIAN_POINT('',(5.5,-1.75,2.));
#7636=CARTESIAN_POINT('',(5.5,-1.75,5.));
#7637=CARTESIAN_POINT('',(5.5,-1.75,5.));
#7638=CARTESIAN_POINT('',(5.5,-1.75,2.));
#7639=CARTESIAN_POINT('Origin',(-5.5,-1.75,2.));
#7640=CARTESIAN_POINT('',(-5.5,-1.75,2.));
#7641=CARTESIAN_POINT('',(-5.5,-1.75,2.));
#7642=CARTESIAN_POINT('',(-5.5,-1.75,5.));
#7643=CARTESIAN_POINT('',(-5.5,-1.75,5.));
#7644=CARTESIAN_POINT('',(-5.5,-1.75,2.));
#7645=CARTESIAN_POINT('Origin',(-5.5,1.75,2.));
#7646=CARTESIAN_POINT('',(-5.5,1.75,2.));
#7647=CARTESIAN_POINT('',(-5.5,1.75,5.));
#7648=CARTESIAN_POINT('Origin',(0.,0.,5.));
#7649=CARTESIAN_POINT('Origin',(0.,0.,2.));
#8225=UNCERTAINTY_MEASURE_WITH_UNIT(LENGTH_MEASURE(0.001),#8267,
'DISTANCE_ACCURACY_VALUE',
'Maximum model space distance between geometric entities at asserted c
onnectivities');
#8241=UNCERTAINTY_MEASURE_WITH_UNIT(LENGTH_MEASURE(0.001),#8267,
'DISTANCE_ACCURACY_VALUE',
'Maximum model space distance between geometric entities at asserted c
onnectivities');
#8250=(
GEOMETRIC_REPRESENTATION_CONTEXT(3)
GLOBAL_UNCERTAINTY_ASSIGNED_CONTEXT((#8225))
GLOBAL_UNIT_ASSIGNED_CONTEXT((#8267,#8269,#8270))
REPRESENTATION_CONTEXT('','3D')
);
#8266=(
GEOMETRIC_REPRESENTATION_CONTEXT(3)
GLOBAL_UNCERTAINTY_ASSIGNED_CONTEXT((#8241))
GLOBAL_UNIT_ASSIGNED_CONTEXT((#8267,#8269,#8270))
REPRESENTATION_CONTEXT('','3D')
);
#8267=(
LENGTH_UNIT()
NAMED_UNIT(*)
SI_UNIT(.CENTI.,.METRE.)
);
#8269=(
NAMED_UNIT(*)
PLANE_ANGLE_UNIT()
SI_UNIT($,.RADIAN.)
);
#8270=(
NAMED_UNIT(*)
SI_UNIT($,.STERADIAN.)
SOLID_ANGLE_UNIT()
);
#8279=SHAPE_DEFINITION_REPRESENTATION(#8303,#8366);
#8303=PRODUCT_DEFINITION_SHAPE('',$,#8391);
#8366=SHAPE_REPRESENTATION('',(#5039),#8250);
#8382=PRODUCT_DEFINITION_CONTEXT('part definition',#8456,'design');
#8391=PRODUCT_DEFINITION('Manifold block','Manifold block',#8415,
#8382);
#8415=PRODUCT_DEFINITION_FORMATION('',$,#8466);
#8456=APPLICATION_CONTEXT(
'Core Data for Automotive Mechanical Design Process');
#8457=PRODUCT_CONTEXT('part definition',#8456,'mechanical');
#8466=PRODUCT('Manifold block','Manifold block',
'Manifold block',(#8457));
#8510=COLOUR_RGB('Dark Blue',0.08,0.2,0.34);
#8511=FILL_AREA_STYLE_COLOUR('',#8510);
#8512=FILL_AREA_STYLE('',(#8511));
#8513=SURFACE_STYLE_FILL_AREA(#8512);
#8514=SURFACE_SIDE_STYLE('',(#8513));
#8515=SURFACE_STYLE_USAGE(.BOTH.,#8514);
#8516=PRESENTATION_STYLE_ASSIGNMENT((#8515));
ENDSEC;
END-ISO-10303-21;
